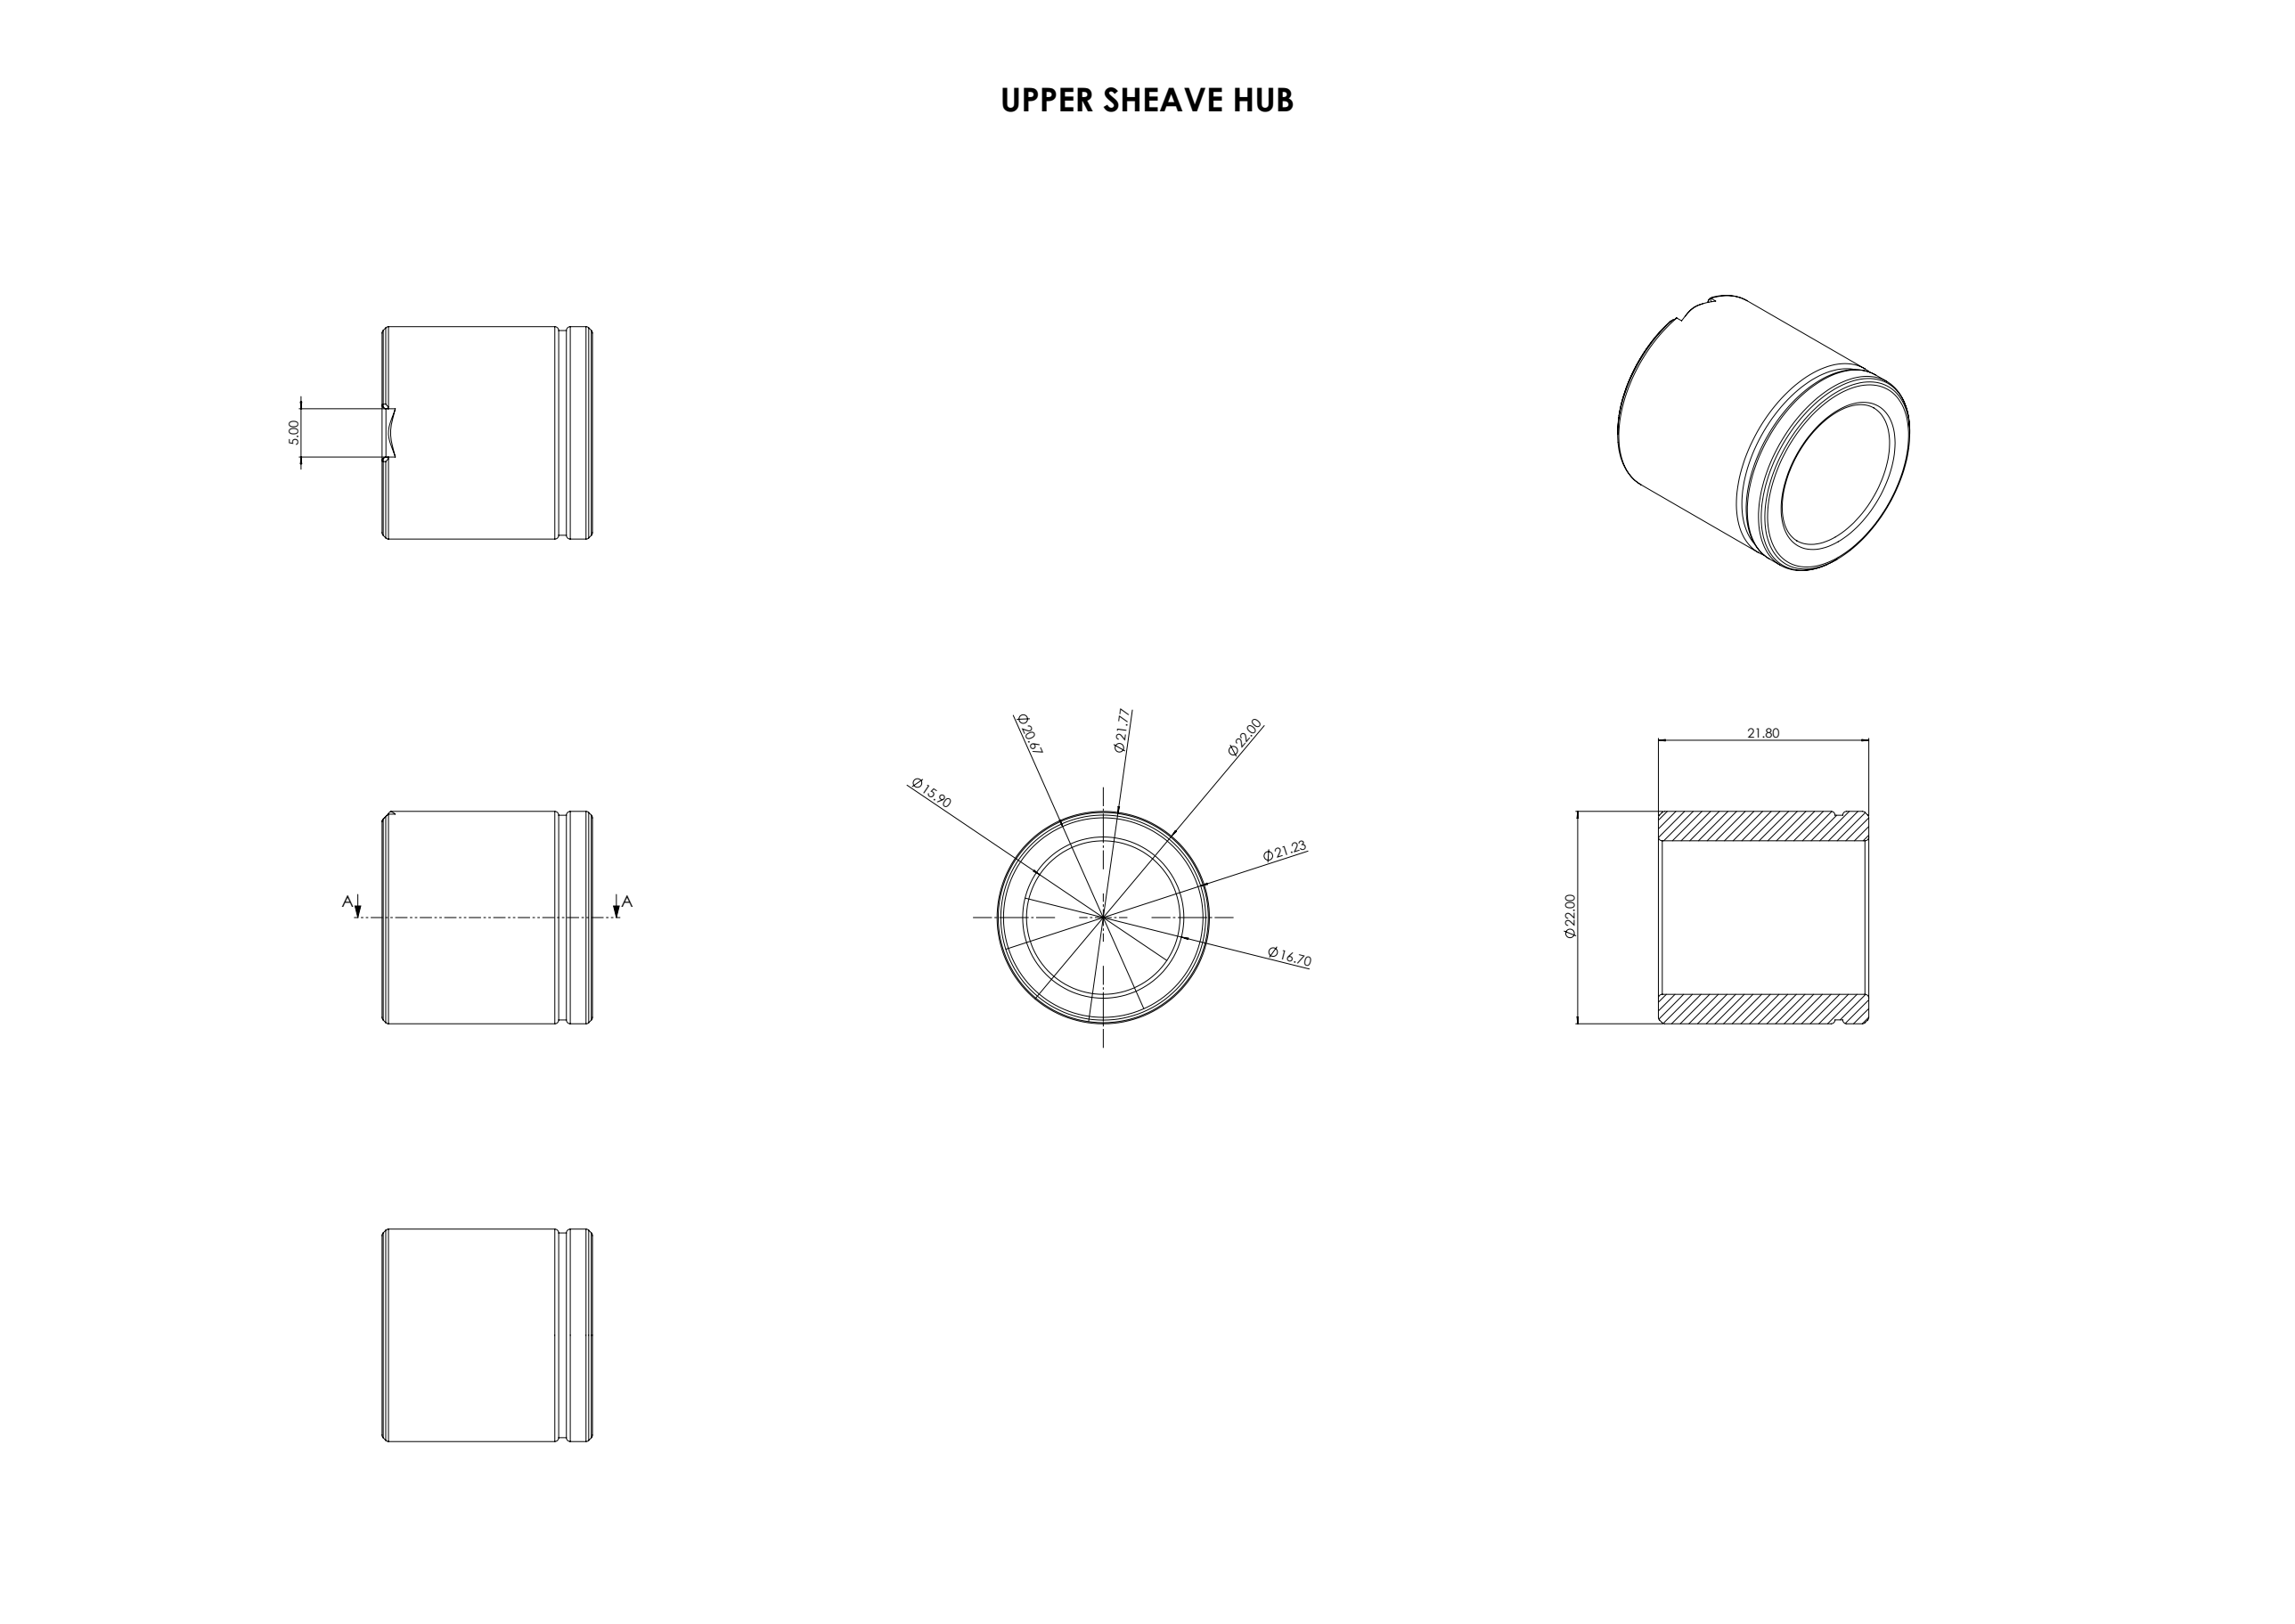
ISO-10303-21;
HEADER;
/* Generated by software containing ST-Developer
 * from STEP Tools, Inc. (www.steptools.com) 
 */

FILE_DESCRIPTION(
/* description */ (''),
/* implementation_level */ '2;1');

FILE_NAME(
/* name */ '05_Upper_Sheave_Hub.step',
/* time_stamp */ '2026-10-24T13:41:11-07:00',
/* author */ (''),
/* organization */ (''),
/* preprocessor_version */ 'ST-DEVELOPER v20.2',
/* originating_system */ 'Autodesk Translation Framework v15.15.0.0',
/* authorisation */ '');

FILE_SCHEMA (('AUTOMOTIVE_DESIGN { 1 0 10303 214 3 1 1 }'));
ENDSEC;

DATA;
#10=MECHANICAL_DESIGN_GEOMETRIC_PRESENTATION_REPRESENTATION('',(#125),#12813);
#77=SPHERICAL_SURFACE('',#4848,0.4);
#78=SPHERICAL_SURFACE('',#4850,0.4);
#79=SPHERICAL_SURFACE('',#4873,0.4);
#80=SPHERICAL_SURFACE('',#4876,0.4);
#92=CONICAL_SURFACE('',#4797,12.45,0.785398163397445);
#93=CONICAL_SURFACE('',#4806,12.45,0.785398163397445);
#94=CONICAL_SURFACE('',#4828,10.75,0.785398163397451);
#95=CONICAL_SURFACE('',#4840,10.75,0.785398163397451);
#105=SHAPE_REPRESENTATION_RELATIONSHIP('SRR','None',#12858,#115);
#115=ADVANCED_BREP_SHAPE_REPRESENTATION('',(#135),#12807);
#125=STYLED_ITEM('',(#12960),#135);
#135=MANIFOLD_SOLID_BREP('Body1',#4388);
#156=FACE_BOUND('',#779,.T.);
#157=FACE_BOUND('',#782,.T.);
#158=FACE_BOUND('',#811,.T.);
#206=PLANE('',#4804);
#207=PLANE('',#4808);
#208=PLANE('',#4816);
#209=PLANE('',#4817);
#210=PLANE('',#4818);
#211=PLANE('',#4819);
#212=PLANE('',#4820);
#213=PLANE('',#4852);
#214=PLANE('',#4855);
#215=PLANE('',#4862);
#216=PLANE('',#4872);
#217=PLANE('',#4884);
#277=TOROIDAL_SURFACE('',#4821,10.6,0.4);
#278=TOROIDAL_SURFACE('',#4831,10.6,0.4);
#279=TOROIDAL_SURFACE('',#4838,10.6,0.4);
#280=TOROIDAL_SURFACE('',#4844,10.3343145750508,0.4);
#281=TOROIDAL_SURFACE('',#4859,10.3343145750508,0.4);
#282=TOROIDAL_SURFACE('',#4864,8.35,0.4);
#283=TOROIDAL_SURFACE('',#4879,8.35,0.4);
#284=TOROIDAL_SURFACE('',#4881,8.35,0.4);
#319=B_SPLINE_SURFACE_WITH_KNOTS('',3,3,((#11947,#11948,#11949,#11950,#11951,
#11952,#11953,#11954,#11955,#11956,#11957,#11958,#11959),(#11960,#11961,
#11962,#11963,#11964,#11965,#11966,#11967,#11968,#11969,#11970,#11971,#11972),
(#11973,#11974,#11975,#11976,#11977,#11978,#11979,#11980,#11981,#11982,
#11983,#11984,#11985),(#11986,#11987,#11988,#11989,#11990,#11991,#11992,
#11993,#11994,#11995,#11996,#11997,#11998),(#11999,#12000,#12001,#12002,
#12003,#12004,#12005,#12006,#12007,#12008,#12009,#12010,#12011),(#12012,
#12013,#12014,#12015,#12016,#12017,#12018,#12019,#12020,#12021,#12022,#12023,
#12024),(#12025,#12026,#12027,#12028,#12029,#12030,#12031,#12032,#12033,
#12034,#12035,#12036,#12037)),.UNSPECIFIED.,.F.,.F.,.F.,(4,1,1,1,4),(4,
1,1,1,1,1,1,1,1,1,4),(0.,0.285714285714286,0.571428571428571,0.785714285714286,
1.),(-0.510305664677257,-0.435654171543958,-0.361002678410658,-0.323676931844009,
-0.305014058560684,-0.286351185277359,-0.267688311994034,-0.211699692144059,
-0.13704819901076,-0.0623967058774603,0.0122547872558393),.UNSPECIFIED.);
#320=B_SPLINE_SURFACE_WITH_KNOTS('',3,3,((#12242,#12243,#12244,#12245),
(#12246,#12247,#12248,#12249),(#12250,#12251,#12252,#12253),(#12254,#12255,
#12256,#12257),(#12258,#12259,#12260,#12261),(#12262,#12263,#12264,#12265)),
 .UNSPECIFIED.,.F.,.F.,.F.,(4,1,1,4),(4,4),(0.,0.285714285714286,0.571428571428571,
1.),(0.,0.0695988259914621),.UNSPECIFIED.);
#321=B_SPLINE_SURFACE_WITH_KNOTS('',3,3,((#12295,#12296,#12297,#12298),
(#12299,#12300,#12301,#12302),(#12303,#12304,#12305,#12306),(#12307,#12308,
#12309,#12310),(#12311,#12312,#12313,#12314)),.UNSPECIFIED.,.F.,.F.,.F.,
(4,1,4),(4,4),(0.248288368736695,0.460547516100694,0.743559712586026),(1.50567154478811,
1.5257178645514),.UNSPECIFIED.);
#322=B_SPLINE_SURFACE_WITH_KNOTS('',3,3,((#12315,#12316,#12317,#12318),
(#12319,#12320,#12321,#12322),(#12323,#12324,#12325,#12326),(#12327,#12328,
#12329,#12330),(#12331,#12332,#12333,#12334)),.UNSPECIFIED.,.F.,.F.,.F.,
(4,1,4),(4,4),(0.248288368736683,0.460547516100081,0.743559712584612),(0.999225034210935,
1.01926765266779),.UNSPECIFIED.);
#323=B_SPLINE_SURFACE_WITH_KNOTS('',3,3,((#12395,#12396,#12397,#12398),
(#12399,#12400,#12401,#12402),(#12403,#12404,#12405,#12406),(#12407,#12408,
#12409,#12410),(#12411,#12412,#12413,#12414),(#12415,#12416,#12417,#12418)),
 .UNSPECIFIED.,.F.,.F.,.F.,(4,1,1,4),(4,4),(0.,0.285714285714286,0.571428571428571,
1.),(0.096109917502246,0.165708743493706),.UNSPECIFIED.);
#491=FACE_OUTER_BOUND('',#776,.T.);
#492=FACE_OUTER_BOUND('',#777,.T.);
#493=FACE_OUTER_BOUND('',#778,.T.);
#494=FACE_OUTER_BOUND('',#780,.T.);
#495=FACE_OUTER_BOUND('',#781,.T.);
#496=FACE_OUTER_BOUND('',#783,.T.);
#497=FACE_OUTER_BOUND('',#784,.T.);
#498=FACE_OUTER_BOUND('',#785,.T.);
#499=FACE_OUTER_BOUND('',#786,.T.);
#500=FACE_OUTER_BOUND('',#787,.T.);
#501=FACE_OUTER_BOUND('',#788,.T.);
#502=FACE_OUTER_BOUND('',#789,.T.);
#503=FACE_OUTER_BOUND('',#790,.T.);
#504=FACE_OUTER_BOUND('',#791,.T.);
#505=FACE_OUTER_BOUND('',#792,.T.);
#506=FACE_OUTER_BOUND('',#793,.T.);
#507=FACE_OUTER_BOUND('',#794,.T.);
#508=FACE_OUTER_BOUND('',#795,.T.);
#509=FACE_OUTER_BOUND('',#796,.T.);
#510=FACE_OUTER_BOUND('',#797,.T.);
#511=FACE_OUTER_BOUND('',#798,.T.);
#512=FACE_OUTER_BOUND('',#799,.T.);
#513=FACE_OUTER_BOUND('',#800,.T.);
#514=FACE_OUTER_BOUND('',#801,.T.);
#515=FACE_OUTER_BOUND('',#802,.T.);
#516=FACE_OUTER_BOUND('',#803,.T.);
#517=FACE_OUTER_BOUND('',#804,.T.);
#518=FACE_OUTER_BOUND('',#805,.T.);
#519=FACE_OUTER_BOUND('',#806,.T.);
#520=FACE_OUTER_BOUND('',#807,.T.);
#521=FACE_OUTER_BOUND('',#808,.T.);
#522=FACE_OUTER_BOUND('',#809,.T.);
#523=FACE_OUTER_BOUND('',#810,.T.);
#524=FACE_OUTER_BOUND('',#812,.T.);
#525=FACE_OUTER_BOUND('',#813,.T.);
#526=FACE_OUTER_BOUND('',#814,.T.);
#527=FACE_OUTER_BOUND('',#815,.T.);
#528=FACE_OUTER_BOUND('',#816,.T.);
#529=FACE_OUTER_BOUND('',#817,.T.);
#530=FACE_OUTER_BOUND('',#818,.T.);
#531=FACE_OUTER_BOUND('',#819,.T.);
#532=FACE_OUTER_BOUND('',#820,.T.);
#533=FACE_OUTER_BOUND('',#821,.T.);
#776=EDGE_LOOP('',(#3569,#3570,#3571,#3572,#3573));
#777=EDGE_LOOP('',(#3574,#3575,#3576,#3577,#3578,#3579));
#778=EDGE_LOOP('',(#3580));
#779=EDGE_LOOP('',(#3581));
#780=EDGE_LOOP('',(#3582,#3583,#3584,#3585,#3586));
#781=EDGE_LOOP('',(#3587));
#782=EDGE_LOOP('',(#3588));
#783=EDGE_LOOP('',(#3589,#3590,#3591,#3592));
#784=EDGE_LOOP('',(#3593,#3594,#3595,#3596));
#785=EDGE_LOOP('',(#3597,#3598,#3599));
#786=EDGE_LOOP('',(#3600,#3601,#3602));
#787=EDGE_LOOP('',(#3603,#3604,#3605));
#788=EDGE_LOOP('',(#3606,#3607,#3608));
#789=EDGE_LOOP('',(#3609,#3610,#3611,#3612,#3613,#3614,#3615,#3616,#3617,
#3618,#3619,#3620,#3621,#3622));
#790=EDGE_LOOP('',(#3623,#3624,#3625,#3626));
#791=EDGE_LOOP('',(#3627,#3628,#3629,#3630,#3631,#3632));
#792=EDGE_LOOP('',(#3633,#3634,#3635,#3636,#3637));
#793=EDGE_LOOP('',(#3638,#3639,#3640,#3641,#3642,#3643));
#794=EDGE_LOOP('',(#3644,#3645,#3646,#3647,#3648));
#795=EDGE_LOOP('',(#3649,#3650,#3651,#3652,#3653,#3654,#3655,#3656,#3657));
#796=EDGE_LOOP('',(#3658,#3659,#3660,#3661,#3662,#3663,#3664,#3665,#3666));
#797=EDGE_LOOP('',(#3667,#3668,#3669,#3670));
#798=EDGE_LOOP('',(#3671,#3672,#3673,#3674,#3675));
#799=EDGE_LOOP('',(#3676,#3677,#3678));
#800=EDGE_LOOP('',(#3679,#3680,#3681));
#801=EDGE_LOOP('',(#3682,#3683,#3684,#3685,#3686));
#802=EDGE_LOOP('',(#3687,#3688,#3689,#3690));
#803=EDGE_LOOP('',(#3691,#3692,#3693));
#804=EDGE_LOOP('',(#3694,#3695,#3696));
#805=EDGE_LOOP('',(#3697,#3698,#3699,#3700,#3701,#3702,#3703,#3704,#3705,
#3706,#3707,#3708,#3709,#3710));
#806=EDGE_LOOP('',(#3711,#3712,#3713,#3714));
#807=EDGE_LOOP('',(#3715,#3716,#3717,#3718));
#808=EDGE_LOOP('',(#3719,#3720,#3721,#3722));
#809=EDGE_LOOP('',(#3723,#3724,#3725,#3726,#3727));
#810=EDGE_LOOP('',(#3728));
#811=EDGE_LOOP('',(#3729));
#812=EDGE_LOOP('',(#3730,#3731,#3732,#3733,#3734));
#813=EDGE_LOOP('',(#3735,#3736,#3737,#3738,#3739,#3740,#3741,#3742,#3743));
#814=EDGE_LOOP('',(#3744,#3745,#3746,#3747,#3748,#3749,#3750,#3751,#3752,
#3753,#3754,#3755));
#815=EDGE_LOOP('',(#3756,#3757,#3758));
#816=EDGE_LOOP('',(#3759,#3760,#3761));
#817=EDGE_LOOP('',(#3762,#3763,#3764,#3765,#3766));
#818=EDGE_LOOP('',(#3767,#3768,#3769,#3770));
#819=EDGE_LOOP('',(#3771,#3772,#3773,#3774,#3775,#3776));
#820=EDGE_LOOP('',(#3777,#3778,#3779,#3780));
#821=EDGE_LOOP('',(#3781,#3782,#3783,#3784));
#1032=CIRCLE('',#4798,12.6);
#1033=CIRCLE('',#4799,12.6);
#1034=CIRCLE('',#4800,12.3);
#1035=CIRCLE('',#4802,12.6);
#1036=CIRCLE('',#4803,12.6);
#1037=CIRCLE('',#4805,10.6);
#1038=CIRCLE('',#4807,12.3);
#1039=CIRCLE('',#4809,11.);
#1040=CIRCLE('',#4811,10.5);
#1041=CIRCLE('',#4812,10.5);
#1042=CIRCLE('',#4814,10.5);
#1043=CIRCLE('',#4815,10.5);
#1044=CIRCLE('',#4822,10.8828427124746);
#1045=CIRCLE('',#4823,10.8828427124746);
#1046=CIRCLE('',#4824,0.4);
#1047=CIRCLE('',#4825,11.);
#1048=CIRCLE('',#4826,11.);
#1049=CIRCLE('',#4829,10.6171572875254);
#1050=CIRCLE('',#4830,10.6171572875254);
#1051=CIRCLE('',#4832,0.4);
#1052=CIRCLE('',#4833,11.);
#1053=CIRCLE('',#4834,11.);
#1054=CIRCLE('',#4836,11.);
#1055=CIRCLE('',#4837,11.);
#1056=CIRCLE('',#4839,10.8828427124746);
#1057=CIRCLE('',#4841,10.6171572875254);
#1058=CIRCLE('',#4842,0.4);
#1059=CIRCLE('',#4843,0.4);
#1060=CIRCLE('',#4845,0.400000000000002);
#1061=CIRCLE('',#4846,10.3343145750508);
#1062=CIRCLE('',#4847,0.4);
#1063=CIRCLE('',#4849,0.400000000000003);
#1064=CIRCLE('',#4851,0.400000000000003);
#1065=CIRCLE('',#4854,0.4);
#1066=CIRCLE('',#4856,8.35);
#1067=CIRCLE('',#4858,0.4);
#1068=CIRCLE('',#4860,10.3343145750508);
#1069=CIRCLE('',#4861,0.4);
#1070=CIRCLE('',#4863,8.35);
#1071=CIRCLE('',#4865,7.95);
#1072=CIRCLE('',#4866,7.95);
#1073=CIRCLE('',#4867,0.4);
#1074=CIRCLE('',#4869,7.95);
#1075=CIRCLE('',#4870,7.95);
#1076=CIRCLE('',#4871,7.95);
#1077=CIRCLE('',#4874,0.4);
#1078=CIRCLE('',#4875,0.4);
#1079=CIRCLE('',#4877,0.400000000000001);
#1080=CIRCLE('',#4878,0.4);
#1081=CIRCLE('',#4882,8.35);
#1236=LINE('',#11795,#1466);
#1237=LINE('',#11802,#1467);
#1238=LINE('',#11809,#1468);
#1239=LINE('',#11816,#1469);
#1240=LINE('',#11820,#1470);
#1241=LINE('',#11825,#1471);
#1242=LINE('',#11829,#1472);
#1243=LINE('',#11833,#1473);
#1244=LINE('',#11834,#1474);
#1245=LINE('',#11837,#1475);
#1246=LINE('',#11838,#1476);
#1247=LINE('',#11841,#1477);
#1248=LINE('',#11842,#1478);
#1249=LINE('',#11845,#1479);
#1250=LINE('',#11846,#1480);
#1251=LINE('',#11849,#1481);
#1252=LINE('',#11851,#1482);
#1253=LINE('',#11858,#1483);
#1254=LINE('',#11860,#1484);
#1255=LINE('',#11901,#1485);
#1256=LINE('',#11946,#1486);
#1257=LINE('',#12141,#1487);
#1258=LINE('',#12146,#1488);
#1259=LINE('',#12156,#1489);
#1260=LINE('',#12159,#1490);
#1261=LINE('',#12436,#1491);
#1262=LINE('',#12438,#1492);
#1263=LINE('',#12440,#1493);
#1264=LINE('',#12447,#1494);
#1265=LINE('',#12448,#1495);
#1266=LINE('',#12451,#1496);
#1267=LINE('',#12455,#1497);
#1268=LINE('',#12474,#1498);
#1269=LINE('',#12478,#1499);
#1270=LINE('',#12482,#1500);
#1271=LINE('',#12485,#1501);
#1466=VECTOR('',#5707,12.45);
#1467=VECTOR('',#5716,12.6);
#1468=VECTOR('',#5725,12.45);
#1469=VECTOR('',#5732,10.);
#1470=VECTOR('',#5735,10.);
#1471=VECTOR('',#5740,10.);
#1472=VECTOR('',#5743,10.);
#1473=VECTOR('',#5748,10.);
#1474=VECTOR('',#5749,10.);
#1475=VECTOR('',#5752,10.);
#1476=VECTOR('',#5753,10.);
#1477=VECTOR('',#5756,10.);
#1478=VECTOR('',#5757,10.);
#1479=VECTOR('',#5760,10.);
#1480=VECTOR('',#5761,10.);
#1481=VECTOR('',#5764,10.);
#1482=VECTOR('',#5765,10.);
#1483=VECTOR('',#5766,10.);
#1484=VECTOR('',#5767,10.);
#1485=VECTOR('',#5768,10.);
#1486=VECTOR('',#5769,10.);
#1487=VECTOR('',#5784,11.);
#1488=VECTOR('',#5789,10.75);
#1489=VECTOR('',#5802,11.);
#1490=VECTOR('',#5805,10.);
#1491=VECTOR('',#5838,10.);
#1492=VECTOR('',#5839,10.);
#1493=VECTOR('',#5840,10.);
#1494=VECTOR('',#5841,10.);
#1495=VECTOR('',#5842,10.);
#1496=VECTOR('',#5845,10.);
#1497=VECTOR('',#5850,10.);
#1498=VECTOR('',#5877,7.95);
#1499=VECTOR('',#5880,10.);
#1500=VECTOR('',#5883,10.);
#1501=VECTOR('',#5888,10.);
#1723=B_SPLINE_CURVE_WITH_KNOTS('',3,(#11853,#11854,#11855,#11856),
 .UNSPECIFIED.,.F.,.F.,(4,4),(-0.0736302548927899,-0.0606102871491874),
 .UNSPECIFIED.);
#1724=B_SPLINE_CURVE_WITH_KNOTS('',3,(#11862,#11863,#11864,#11865),
 .UNSPECIFIED.,.F.,.F.,(4,4),(-0.0535503409172659,0.),.UNSPECIFIED.);
#1725=B_SPLINE_CURVE_WITH_KNOTS('',3,(#11867,#11868,#11869,#11870,#11871,
#11872,#11873,#11874,#11875,#11876,#11877,#11878,#11879,#11880,#11881,#11882,
#11883,#11884,#11885,#11886,#11887,#11888,#11889,#11890,#11891,#11892,#11893,
#11894),.UNSPECIFIED.,.F.,.F.,(4,3,3,3,3,3,3,3,3,4),(-0.0707543141709639,
-0.0639700558869814,-0.0618906129072222,-0.0551601393419019,-0.0506565173110961,
-0.0464091777054624,-0.039691133709109,-0.0329985150203425,-0.0311186796527011,
-0.0241191350787041),.UNSPECIFIED.);
#1726=B_SPLINE_CURVE_WITH_KNOTS('',3,(#11896,#11897,#11898,#11899),
 .UNSPECIFIED.,.F.,.F.,(4,4),(0.,0.00710537445304894),.UNSPECIFIED.);
#1727=B_SPLINE_CURVE_WITH_KNOTS('',3,(#11903,#11904,#11905,#11906,#11907,
#11908,#11909,#11910,#11911,#11912,#11913,#11914,#11915,#11916,#11917,#11918,
#11919,#11920,#11921,#11922,#11923,#11924,#11925,#11926,#11927,#11928,#11929,
#11930,#11931,#11932,#11933,#11934,#11935,#11936,#11937,#11938,#11939,#11940,
#11941,#11942,#11943,#11944,#11945),.UNSPECIFIED.,.F.,.F.,(4,3,3,3,3,3,
3,3,3,3,3,3,3,3,4),(0.,0.00580629857172819,0.011668120368983,0.0175829585474277,
0.0201349204647166,0.0268347020686461,0.0295682026475181,0.0365019513209761,
0.0408129765218727,0.0451592379215555,0.0520962433453293,0.0563360701356979,
0.0584849555420972,0.0655164894020243,0.0715864535936182),.UNSPECIFIED.);
#1728=B_SPLINE_CURVE_WITH_KNOTS('',3,(#12040,#12041,#12042,#12043,#12044,
#12045,#12046,#12047,#12048,#12049,#12050,#12051,#12052,#12053,#12054,#12055,
#12056,#12057,#12058,#12059,#12060,#12061,#12062,#12063,#12064,#12065,#12066,
#12067,#12068,#12069,#12070,#12071,#12072,#12073,#12074,#12075,#12076,#12077,
#12078,#12079,#12080,#12081,#12082,#12083,#12084,#12085),.UNSPECIFIED.,
 .F.,.F.,(4,3,3,3,3,3,3,3,3,3,3,3,3,3,3,4),(0.,0.00694526795998421,0.0139543072598735,
0.015291136260988,0.0172103975930811,0.0240884241491964,0.0308533616756733,
0.0340363892002112,0.0409613583285485,0.0476241304298719,0.0499527776364528,
0.0515655803640436,0.0584478624259065,0.0609496822139948,0.0675796538345217,
0.0717651027806449),.UNSPECIFIED.);
#1729=B_SPLINE_CURVE_WITH_KNOTS('',3,(#12086,#12087,#12088,#12089,#12090,
#12091,#12092,#12093,#12094,#12095,#12096,#12097,#12098),.UNSPECIFIED.,
 .F.,.F.,(4,1,1,1,1,1,1,1,1,1,4),(-0.0122547872558393,0.0623967058774603,
0.13704819901076,0.211699692144059,0.267688311994034,0.286351185277359,
0.305014058560684,0.323676931844009,0.361002678410658,0.435654171543958,
0.510305664677257),.UNSPECIFIED.);
#1730=B_SPLINE_CURVE_WITH_KNOTS('',3,(#12099,#12100,#12101,#12102,#12103,
#12104,#12105,#12106,#12107,#12108,#12109,#12110,#12111,#12112,#12113,#12114,
#12115,#12116,#12117,#12118,#12119,#12120,#12121,#12122,#12123,#12124,#12125,
#12126,#12127,#12128,#12129),.UNSPECIFIED.,.F.,.F.,(4,3,3,3,3,3,3,3,3,3,
4),(0.000383354128218201,0.0625597845796719,0.136949375128678,0.174144170403181,
0.192741568040432,0.211338965677684,0.229936363314935,0.28572855622669,
0.360118146775696,0.434507737324702,0.496685534539592),.UNSPECIFIED.);
#1731=B_SPLINE_CURVE_WITH_KNOTS('',3,(#12163,#12164,#12165,#12166),
 .UNSPECIFIED.,.F.,.F.,(4,4),(-0.00710537445449871,0.),.UNSPECIFIED.);
#1732=B_SPLINE_CURVE_WITH_KNOTS('',3,(#12168,#12169,#12170,#12171),
 .UNSPECIFIED.,.F.,.F.,(4,4),(-0.0196379557516152,-0.000110621155015422),
 .UNSPECIFIED.);
#1733=B_SPLINE_CURVE_WITH_KNOTS('',3,(#12173,#12174,#12175,#12176,#12177,
#12178,#12179,#12180,#12181,#12182,#12183,#12184,#12185,#12186,#12187,#12188,
#12189,#12190,#12191,#12192,#12193,#12194,#12195,#12196,#12197),
 .UNSPECIFIED.,.F.,.F.,(4,3,3,3,3,3,3,3,4),(-0.0420242349144714,-0.034244024011145,
-0.0304445564291344,-0.0224018409775603,-0.0210691966450077,-0.0115168785817897,
-0.00144892293139089,0.,0.000288034171025875),.UNSPECIFIED.);
#1734=B_SPLINE_CURVE_WITH_KNOTS('',3,(#12201,#12202,#12203,#12204,#12205,
#12206,#12207,#12208,#12209,#12210,#12211,#12212,#12213,#12214,#12215,#12216,
#12217,#12218,#12219,#12220,#12221,#12222,#12223,#12224,#12225),
 .UNSPECIFIED.,.F.,.F.,(4,3,3,3,3,3,3,3,4),(-0.0422600918508368,-0.0419734950304658,
-0.0314914666110231,-0.021986817507206,-0.0210094381915805,-0.01300685760943,
-0.0116808634569233,-0.00393947746920935,-0.000158970042657082),
 .UNSPECIFIED.);
#1735=B_SPLINE_CURVE_WITH_KNOTS('',3,(#12226,#12227,#12228,#12229),
 .UNSPECIFIED.,.F.,.F.,(4,4),(-0.328977585058273,-0.317010469451376),
 .UNSPECIFIED.);
#1736=B_SPLINE_CURVE_WITH_KNOTS('',3,(#12232,#12233,#12234,#12235),
 .UNSPECIFIED.,.F.,.F.,(4,4),(0.,0.0383467777019652),.UNSPECIFIED.);
#1737=B_SPLINE_CURVE_WITH_KNOTS('',3,(#12238,#12239,#12240,#12241),
 .UNSPECIFIED.,.F.,.F.,(4,4),(0.127361965791744,0.165708743493706),
 .UNSPECIFIED.);
#1738=B_SPLINE_CURVE_WITH_KNOTS('',3,(#12266,#12267,#12268,#12269,#12270,
#12271,#12272,#12273,#12274,#12275,#12276,#12277,#12278,#12279,#12280,#12281,
#12282,#12283,#12284,#12285,#12286,#12287,#12288,#12289,#12290,#12291,#12292,
#12293),.UNSPECIFIED.,.F.,.F.,(4,3,3,3,3,3,3,3,3,4),(-0.103312994452742,
-0.0944972367595641,-0.0896726356037232,-0.081979706066035,-0.0758675452743191,
-0.0681010871890584,-0.0620124392214268,-0.0585654250906251,-0.0490657070288485,
-0.0435218377980582),.UNSPECIFIED.);
#1739=B_SPLINE_CURVE_WITH_KNOTS('',3,(#12336,#12337,#12338,#12339,#12340,
#12341,#12342,#12343,#12344,#12345,#12346,#12347,#12348,#12349,#12350,#12351,
#12352,#12353,#12354,#12355,#12356,#12357,#12358,#12359,#12360,#12361,#12362,
#12363,#12364,#12365,#12366),.UNSPECIFIED.,.F.,.F.,(4,3,3,3,3,3,3,3,3,3,
4),(-0.0462738036441523,-0.0389589150096727,-0.0346312122739206,-0.0286583377057116,
-0.0230059035179827,-0.0212406883770576,-0.0202962772284038,-0.014379131563933,
-0.0105565993757205,-0.00393990817803328,0.),.UNSPECIFIED.);
#1740=B_SPLINE_CURVE_WITH_KNOTS('',3,(#12367,#12368,#12369,#12370,#12371,
#12372,#12373,#12374,#12375,#12376,#12377,#12378,#12379,#12380,#12381,#12382,
#12383,#12384,#12385,#12386,#12387,#12388,#12389,#12390,#12391,#12392,#12393,
#12394),.UNSPECIFIED.,.F.,.F.,(4,3,3,3,3,3,3,3,3,4),(-0.070410764499354,
-0.0637409419809624,-0.0570604470106178,-0.0503274465588287,-0.0483425491955468,
-0.0438577936617308,-0.0371215088649918,-0.0325914562918353,-0.0258040649471257,
-0.023746438679814),.UNSPECIFIED.);
#1741=B_SPLINE_CURVE_WITH_KNOTS('',3,(#12421,#12422,#12423,#12424),
 .UNSPECIFIED.,.F.,.F.,(4,4),(-0.165708743493706,-0.112158402576443),
 .UNSPECIFIED.);
#1742=B_SPLINE_CURVE_WITH_KNOTS('',3,(#12442,#12443,#12444,#12445),
 .UNSPECIFIED.,.F.,.F.,(4,4),(-0.182084709739034,-0.169064741995431),
 .UNSPECIFIED.);
#1743=B_SPLINE_CURVE_WITH_KNOTS('',3,(#12494,#12495,#12496,#12497,#12498,
#12499,#12500,#12501,#12502,#12503),.UNSPECIFIED.,.F.,.F.,(4,2,2,2,4),(-0.000394703056647228,
0.,0.0306355392027269,0.0540522668896819,0.0684604040501524),
 .UNSPECIFIED.);
#1744=B_SPLINE_CURVE_WITH_KNOTS('',3,(#12505,#12506,#12507,#12508,#12509,
#12510,#12511,#12512,#12513,#12514),.UNSPECIFIED.,.F.,.F.,(4,2,2,2,4),(-0.147143178540475,
-0.1468201126579,-0.121744812771334,-0.102578136276002,-0.0907850237818083),
 .UNSPECIFIED.);
#1996=VERTEX_POINT('',#11790);
#1997=VERTEX_POINT('',#11791);
#1998=VERTEX_POINT('',#11794);
#1999=VERTEX_POINT('',#11798);
#2000=VERTEX_POINT('',#11799);
#2001=VERTEX_POINT('',#11804);
#2002=VERTEX_POINT('',#11807);
#2003=VERTEX_POINT('',#11811);
#2004=VERTEX_POINT('',#11814);
#2005=VERTEX_POINT('',#11815);
#2006=VERTEX_POINT('',#11817);
#2007=VERTEX_POINT('',#11819);
#2008=VERTEX_POINT('',#11823);
#2009=VERTEX_POINT('',#11824);
#2010=VERTEX_POINT('',#11826);
#2011=VERTEX_POINT('',#11828);
#2012=VERTEX_POINT('',#11832);
#2013=VERTEX_POINT('',#11836);
#2014=VERTEX_POINT('',#11840);
#2015=VERTEX_POINT('',#11844);
#2016=VERTEX_POINT('',#11848);
#2017=VERTEX_POINT('',#11850);
#2018=VERTEX_POINT('',#11852);
#2019=VERTEX_POINT('',#11857);
#2020=VERTEX_POINT('',#11859);
#2021=VERTEX_POINT('',#11861);
#2022=VERTEX_POINT('',#11866);
#2023=VERTEX_POINT('',#11895);
#2024=VERTEX_POINT('',#11900);
#2025=VERTEX_POINT('',#11902);
#2026=VERTEX_POINT('',#12038);
#2027=VERTEX_POINT('',#12039);
#2028=VERTEX_POINT('',#12131);
#2029=VERTEX_POINT('',#12132);
#2030=VERTEX_POINT('',#12135);
#2031=VERTEX_POINT('',#12137);
#2032=VERTEX_POINT('',#12143);
#2033=VERTEX_POINT('',#12144);
#2034=VERTEX_POINT('',#12149);
#2035=VERTEX_POINT('',#12151);
#2036=VERTEX_POINT('',#12155);
#2037=VERTEX_POINT('',#12157);
#2038=VERTEX_POINT('',#12162);
#2039=VERTEX_POINT('',#12167);
#2040=VERTEX_POINT('',#12172);
#2041=VERTEX_POINT('',#12198);
#2042=VERTEX_POINT('',#12200);
#2043=VERTEX_POINT('',#12231);
#2044=VERTEX_POINT('',#12236);
#2045=VERTEX_POINT('',#12335);
#2046=VERTEX_POINT('',#12419);
#2047=VERTEX_POINT('',#12426);
#2048=VERTEX_POINT('',#12428);
#2049=VERTEX_POINT('',#12437);
#2050=VERTEX_POINT('',#12439);
#2051=VERTEX_POINT('',#12441);
#2052=VERTEX_POINT('',#12446);
#2053=VERTEX_POINT('',#12450);
#2054=VERTEX_POINT('',#12454);
#2055=VERTEX_POINT('',#12460);
#2056=VERTEX_POINT('',#12464);
#2057=VERTEX_POINT('',#12467);
#2058=VERTEX_POINT('',#12468);
#2059=VERTEX_POINT('',#12473);
#2060=VERTEX_POINT('',#12475);
#2061=VERTEX_POINT('',#12477);
#2062=VERTEX_POINT('',#12479);
#2063=VERTEX_POINT('',#12481);
#2537=EDGE_CURVE('',#1996,#1997,#1032,.T.);
#2538=EDGE_CURVE('',#1997,#1996,#1033,.T.);
#2539=EDGE_CURVE('',#1996,#1998,#1236,.T.);
#2540=EDGE_CURVE('',#1998,#1998,#1034,.T.);
#2541=EDGE_CURVE('',#1999,#2000,#1035,.T.);
#2542=EDGE_CURVE('',#2000,#1999,#1036,.T.);
#2543=EDGE_CURVE('',#2000,#1997,#1237,.T.);
#2544=EDGE_CURVE('',#2001,#2001,#1037,.T.);
#2545=EDGE_CURVE('',#2002,#2002,#1038,.T.);
#2546=EDGE_CURVE('',#2002,#1999,#1238,.T.);
#2547=EDGE_CURVE('',#2003,#2003,#1039,.T.);
#2548=EDGE_CURVE('',#2004,#2005,#1239,.T.);
#2549=EDGE_CURVE('',#2006,#2004,#1040,.T.);
#2550=EDGE_CURVE('',#2007,#2006,#1240,.T.);
#2551=EDGE_CURVE('',#2007,#2005,#1041,.T.);
#2552=EDGE_CURVE('',#2008,#2009,#1241,.T.);
#2553=EDGE_CURVE('',#2008,#2010,#1042,.T.);
#2554=EDGE_CURVE('',#2011,#2010,#1242,.T.);
#2555=EDGE_CURVE('',#2009,#2011,#1043,.T.);
#2556=EDGE_CURVE('',#2005,#2012,#1243,.T.);
#2557=EDGE_CURVE('',#2012,#2007,#1244,.T.);
#2558=EDGE_CURVE('',#2013,#2008,#1245,.T.);
#2559=EDGE_CURVE('',#2010,#2013,#1246,.T.);
#2560=EDGE_CURVE('',#2014,#2004,#1247,.T.);
#2561=EDGE_CURVE('',#2006,#2014,#1248,.T.);
#2562=EDGE_CURVE('',#2009,#2015,#1249,.T.);
#2563=EDGE_CURVE('',#2015,#2011,#1250,.T.);
#2564=EDGE_CURVE('',#2016,#2013,#1251,.T.);
#2565=EDGE_CURVE('',#2017,#2016,#1252,.T.);
#2566=EDGE_CURVE('',#2018,#2017,#1723,.T.);
#2567=EDGE_CURVE('',#2019,#2018,#1253,.T.);
#2568=EDGE_CURVE('',#2020,#2019,#1254,.T.);
#2569=EDGE_CURVE('',#2021,#2020,#1724,.T.);
#2570=EDGE_CURVE('',#2021,#2022,#1725,.T.);
#2571=EDGE_CURVE('',#2023,#2022,#1726,.T.);
#2572=EDGE_CURVE('',#2023,#2024,#1255,.T.);
#2573=EDGE_CURVE('',#2025,#2024,#1727,.F.);
#2574=EDGE_CURVE('',#2015,#2025,#1256,.T.);
#2575=EDGE_CURVE('',#2026,#2027,#1728,.T.);
#2576=EDGE_CURVE('',#2026,#2025,#1729,.T.);
#2577=EDGE_CURVE('',#2024,#2027,#1730,.T.);
#2578=EDGE_CURVE('',#2028,#2029,#1044,.T.);
#2579=EDGE_CURVE('',#2029,#2028,#1045,.T.);
#2580=EDGE_CURVE('',#2028,#2030,#1046,.T.);
#2581=EDGE_CURVE('',#2030,#2031,#1047,.T.);
#2582=EDGE_CURVE('',#2031,#2030,#1048,.T.);
#2583=EDGE_CURVE('',#2031,#2003,#1257,.T.);
#2584=EDGE_CURVE('',#2032,#2033,#1049,.T.);
#2585=EDGE_CURVE('',#2032,#2029,#1258,.T.);
#2586=EDGE_CURVE('',#2033,#2032,#1050,.T.);
#2587=EDGE_CURVE('',#2001,#2034,#1051,.T.);
#2588=EDGE_CURVE('',#2034,#2035,#1052,.T.);
#2589=EDGE_CURVE('',#2035,#2034,#1053,.T.);
#2590=EDGE_CURVE('',#2035,#2036,#1259,.T.);
#2591=EDGE_CURVE('',#2037,#2036,#1054,.T.);
#2592=EDGE_CURVE('',#2027,#2037,#1260,.T.);
#2593=EDGE_CURVE('',#2036,#2023,#1055,.T.);
#2594=EDGE_CURVE('',#2038,#2037,#1731,.T.);
#2595=EDGE_CURVE('',#2022,#2039,#1732,.T.);
#2596=EDGE_CURVE('',#2039,#2040,#1733,.T.);
#2597=EDGE_CURVE('',#2040,#2041,#1056,.T.);
#2598=EDGE_CURVE('',#2041,#2042,#1734,.T.);
#2599=EDGE_CURVE('',#2042,#2038,#1735,.T.);
#2600=EDGE_CURVE('',#2043,#2040,#1736,.T.);
#2601=EDGE_CURVE('',#2044,#2043,#1057,.T.);
#2602=EDGE_CURVE('',#2041,#2044,#1737,.T.);
#2603=EDGE_CURVE('',#2021,#2039,#1738,.T.);
#2604=EDGE_CURVE('',#2020,#2043,#1058,.T.);
#2605=EDGE_CURVE('',#2045,#2042,#1739,.F.);
#2606=EDGE_CURVE('',#2038,#2045,#1740,.T.);
#2607=EDGE_CURVE('',#2044,#2046,#1059,.T.);
#2608=EDGE_CURVE('',#2046,#2045,#1741,.T.);
#2609=EDGE_CURVE('',#2043,#2047,#1060,.T.);
#2610=EDGE_CURVE('',#2047,#2048,#1061,.T.);
#2611=EDGE_CURVE('',#2048,#2044,#1062,.T.);
#2612=EDGE_CURVE('',#2048,#2046,#1063,.T.);
#2613=EDGE_CURVE('',#2020,#2047,#1064,.T.);
#2614=EDGE_CURVE('',#2026,#2014,#1261,.T.);
#2615=EDGE_CURVE('',#2049,#2046,#1262,.T.);
#2616=EDGE_CURVE('',#2050,#2049,#1263,.T.);
#2617=EDGE_CURVE('',#2051,#2050,#1742,.T.);
#2618=EDGE_CURVE('',#2052,#2051,#1264,.T.);
#2619=EDGE_CURVE('',#2012,#2052,#1265,.T.);
#2620=EDGE_CURVE('',#2048,#2053,#1266,.T.);
#2621=EDGE_CURVE('',#2053,#2049,#1065,.F.);
#2622=EDGE_CURVE('',#2054,#2047,#1267,.T.);
#2623=EDGE_CURVE('',#2053,#2054,#1066,.T.);
#2624=EDGE_CURVE('',#2019,#2054,#1067,.F.);
#2625=EDGE_CURVE('',#2055,#2055,#1068,.T.);
#2626=EDGE_CURVE('',#2055,#2033,#1069,.T.);
#2627=EDGE_CURVE('',#2056,#2056,#1070,.T.);
#2628=EDGE_CURVE('',#2057,#2058,#1071,.T.);
#2629=EDGE_CURVE('',#2058,#2057,#1072,.T.);
#2630=EDGE_CURVE('',#2057,#2056,#1073,.T.);
#2631=EDGE_CURVE('',#2058,#2059,#1268,.T.);
#2632=EDGE_CURVE('',#2060,#2059,#1074,.T.);
#2633=EDGE_CURVE('',#2061,#2060,#1269,.T.);
#2634=EDGE_CURVE('',#2062,#2061,#1075,.T.);
#2635=EDGE_CURVE('',#2063,#2062,#1270,.T.);
#2636=EDGE_CURVE('',#2059,#2063,#1076,.T.);
#2637=EDGE_CURVE('',#2052,#2016,#1271,.T.);
#2638=EDGE_CURVE('',#2049,#2063,#1077,.F.);
#2639=EDGE_CURVE('',#2063,#2053,#1078,.F.);
#2640=EDGE_CURVE('',#2060,#2019,#1079,.F.);
#2641=EDGE_CURVE('',#2054,#2060,#1080,.F.);
#2642=EDGE_CURVE('',#2062,#2050,#1743,.T.);
#2643=EDGE_CURVE('',#2061,#2018,#1744,.T.);
#2644=EDGE_CURVE('',#2017,#2051,#1081,.T.);
#3569=ORIENTED_EDGE('',*,*,#2537,.T.);
#3570=ORIENTED_EDGE('',*,*,#2538,.T.);
#3571=ORIENTED_EDGE('',*,*,#2539,.T.);
#3572=ORIENTED_EDGE('',*,*,#2540,.T.);
#3573=ORIENTED_EDGE('',*,*,#2539,.F.);
#3574=ORIENTED_EDGE('',*,*,#2541,.F.);
#3575=ORIENTED_EDGE('',*,*,#2542,.F.);
#3576=ORIENTED_EDGE('',*,*,#2543,.T.);
#3577=ORIENTED_EDGE('',*,*,#2537,.F.);
#3578=ORIENTED_EDGE('',*,*,#2538,.F.);
#3579=ORIENTED_EDGE('',*,*,#2543,.F.);
#3580=ORIENTED_EDGE('',*,*,#2540,.F.);
#3581=ORIENTED_EDGE('',*,*,#2544,.T.);
#3582=ORIENTED_EDGE('',*,*,#2545,.T.);
#3583=ORIENTED_EDGE('',*,*,#2546,.T.);
#3584=ORIENTED_EDGE('',*,*,#2541,.T.);
#3585=ORIENTED_EDGE('',*,*,#2542,.T.);
#3586=ORIENTED_EDGE('',*,*,#2546,.F.);
#3587=ORIENTED_EDGE('',*,*,#2545,.F.);
#3588=ORIENTED_EDGE('',*,*,#2547,.T.);
#3589=ORIENTED_EDGE('',*,*,#2548,.F.);
#3590=ORIENTED_EDGE('',*,*,#2549,.F.);
#3591=ORIENTED_EDGE('',*,*,#2550,.F.);
#3592=ORIENTED_EDGE('',*,*,#2551,.T.);
#3593=ORIENTED_EDGE('',*,*,#2552,.F.);
#3594=ORIENTED_EDGE('',*,*,#2553,.T.);
#3595=ORIENTED_EDGE('',*,*,#2554,.F.);
#3596=ORIENTED_EDGE('',*,*,#2555,.F.);
#3597=ORIENTED_EDGE('',*,*,#2556,.F.);
#3598=ORIENTED_EDGE('',*,*,#2551,.F.);
#3599=ORIENTED_EDGE('',*,*,#2557,.F.);
#3600=ORIENTED_EDGE('',*,*,#2558,.F.);
#3601=ORIENTED_EDGE('',*,*,#2559,.F.);
#3602=ORIENTED_EDGE('',*,*,#2553,.F.);
#3603=ORIENTED_EDGE('',*,*,#2560,.F.);
#3604=ORIENTED_EDGE('',*,*,#2561,.F.);
#3605=ORIENTED_EDGE('',*,*,#2549,.T.);
#3606=ORIENTED_EDGE('',*,*,#2562,.F.);
#3607=ORIENTED_EDGE('',*,*,#2555,.T.);
#3608=ORIENTED_EDGE('',*,*,#2563,.F.);
#3609=ORIENTED_EDGE('',*,*,#2563,.T.);
#3610=ORIENTED_EDGE('',*,*,#2554,.T.);
#3611=ORIENTED_EDGE('',*,*,#2559,.T.);
#3612=ORIENTED_EDGE('',*,*,#2564,.F.);
#3613=ORIENTED_EDGE('',*,*,#2565,.F.);
#3614=ORIENTED_EDGE('',*,*,#2566,.F.);
#3615=ORIENTED_EDGE('',*,*,#2567,.F.);
#3616=ORIENTED_EDGE('',*,*,#2568,.F.);
#3617=ORIENTED_EDGE('',*,*,#2569,.F.);
#3618=ORIENTED_EDGE('',*,*,#2570,.T.);
#3619=ORIENTED_EDGE('',*,*,#2571,.F.);
#3620=ORIENTED_EDGE('',*,*,#2572,.T.);
#3621=ORIENTED_EDGE('',*,*,#2573,.F.);
#3622=ORIENTED_EDGE('',*,*,#2574,.F.);
#3623=ORIENTED_EDGE('',*,*,#2575,.F.);
#3624=ORIENTED_EDGE('',*,*,#2576,.T.);
#3625=ORIENTED_EDGE('',*,*,#2573,.T.);
#3626=ORIENTED_EDGE('',*,*,#2577,.T.);
#3627=ORIENTED_EDGE('',*,*,#2578,.T.);
#3628=ORIENTED_EDGE('',*,*,#2579,.T.);
#3629=ORIENTED_EDGE('',*,*,#2580,.T.);
#3630=ORIENTED_EDGE('',*,*,#2581,.T.);
#3631=ORIENTED_EDGE('',*,*,#2582,.T.);
#3632=ORIENTED_EDGE('',*,*,#2580,.F.);
#3633=ORIENTED_EDGE('',*,*,#2582,.F.);
#3634=ORIENTED_EDGE('',*,*,#2583,.T.);
#3635=ORIENTED_EDGE('',*,*,#2547,.F.);
#3636=ORIENTED_EDGE('',*,*,#2583,.F.);
#3637=ORIENTED_EDGE('',*,*,#2581,.F.);
#3638=ORIENTED_EDGE('',*,*,#2584,.F.);
#3639=ORIENTED_EDGE('',*,*,#2585,.T.);
#3640=ORIENTED_EDGE('',*,*,#2578,.F.);
#3641=ORIENTED_EDGE('',*,*,#2579,.F.);
#3642=ORIENTED_EDGE('',*,*,#2585,.F.);
#3643=ORIENTED_EDGE('',*,*,#2586,.F.);
#3644=ORIENTED_EDGE('',*,*,#2544,.F.);
#3645=ORIENTED_EDGE('',*,*,#2587,.T.);
#3646=ORIENTED_EDGE('',*,*,#2588,.T.);
#3647=ORIENTED_EDGE('',*,*,#2589,.T.);
#3648=ORIENTED_EDGE('',*,*,#2587,.F.);
#3649=ORIENTED_EDGE('',*,*,#2589,.F.);
#3650=ORIENTED_EDGE('',*,*,#2590,.T.);
#3651=ORIENTED_EDGE('',*,*,#2591,.F.);
#3652=ORIENTED_EDGE('',*,*,#2592,.F.);
#3653=ORIENTED_EDGE('',*,*,#2577,.F.);
#3654=ORIENTED_EDGE('',*,*,#2572,.F.);
#3655=ORIENTED_EDGE('',*,*,#2593,.F.);
#3656=ORIENTED_EDGE('',*,*,#2590,.F.);
#3657=ORIENTED_EDGE('',*,*,#2588,.F.);
#3658=ORIENTED_EDGE('',*,*,#2594,.T.);
#3659=ORIENTED_EDGE('',*,*,#2591,.T.);
#3660=ORIENTED_EDGE('',*,*,#2593,.T.);
#3661=ORIENTED_EDGE('',*,*,#2571,.T.);
#3662=ORIENTED_EDGE('',*,*,#2595,.T.);
#3663=ORIENTED_EDGE('',*,*,#2596,.T.);
#3664=ORIENTED_EDGE('',*,*,#2597,.T.);
#3665=ORIENTED_EDGE('',*,*,#2598,.T.);
#3666=ORIENTED_EDGE('',*,*,#2599,.T.);
#3667=ORIENTED_EDGE('',*,*,#2597,.F.);
#3668=ORIENTED_EDGE('',*,*,#2600,.F.);
#3669=ORIENTED_EDGE('',*,*,#2601,.F.);
#3670=ORIENTED_EDGE('',*,*,#2602,.F.);
#3671=ORIENTED_EDGE('',*,*,#2596,.F.);
#3672=ORIENTED_EDGE('',*,*,#2603,.F.);
#3673=ORIENTED_EDGE('',*,*,#2569,.T.);
#3674=ORIENTED_EDGE('',*,*,#2604,.T.);
#3675=ORIENTED_EDGE('',*,*,#2600,.T.);
#3676=ORIENTED_EDGE('',*,*,#2595,.F.);
#3677=ORIENTED_EDGE('',*,*,#2570,.F.);
#3678=ORIENTED_EDGE('',*,*,#2603,.T.);
#3679=ORIENTED_EDGE('',*,*,#2599,.F.);
#3680=ORIENTED_EDGE('',*,*,#2605,.F.);
#3681=ORIENTED_EDGE('',*,*,#2606,.F.);
#3682=ORIENTED_EDGE('',*,*,#2598,.F.);
#3683=ORIENTED_EDGE('',*,*,#2602,.T.);
#3684=ORIENTED_EDGE('',*,*,#2607,.T.);
#3685=ORIENTED_EDGE('',*,*,#2608,.T.);
#3686=ORIENTED_EDGE('',*,*,#2605,.T.);
#3687=ORIENTED_EDGE('',*,*,#2609,.T.);
#3688=ORIENTED_EDGE('',*,*,#2610,.T.);
#3689=ORIENTED_EDGE('',*,*,#2611,.T.);
#3690=ORIENTED_EDGE('',*,*,#2601,.T.);
#3691=ORIENTED_EDGE('',*,*,#2611,.F.);
#3692=ORIENTED_EDGE('',*,*,#2612,.T.);
#3693=ORIENTED_EDGE('',*,*,#2607,.F.);
#3694=ORIENTED_EDGE('',*,*,#2604,.F.);
#3695=ORIENTED_EDGE('',*,*,#2613,.T.);
#3696=ORIENTED_EDGE('',*,*,#2609,.F.);
#3697=ORIENTED_EDGE('',*,*,#2561,.T.);
#3698=ORIENTED_EDGE('',*,*,#2614,.F.);
#3699=ORIENTED_EDGE('',*,*,#2575,.T.);
#3700=ORIENTED_EDGE('',*,*,#2592,.T.);
#3701=ORIENTED_EDGE('',*,*,#2594,.F.);
#3702=ORIENTED_EDGE('',*,*,#2606,.T.);
#3703=ORIENTED_EDGE('',*,*,#2608,.F.);
#3704=ORIENTED_EDGE('',*,*,#2615,.F.);
#3705=ORIENTED_EDGE('',*,*,#2616,.F.);
#3706=ORIENTED_EDGE('',*,*,#2617,.F.);
#3707=ORIENTED_EDGE('',*,*,#2618,.F.);
#3708=ORIENTED_EDGE('',*,*,#2619,.F.);
#3709=ORIENTED_EDGE('',*,*,#2557,.T.);
#3710=ORIENTED_EDGE('',*,*,#2550,.T.);
#3711=ORIENTED_EDGE('',*,*,#2612,.F.);
#3712=ORIENTED_EDGE('',*,*,#2620,.T.);
#3713=ORIENTED_EDGE('',*,*,#2621,.T.);
#3714=ORIENTED_EDGE('',*,*,#2615,.T.);
#3715=ORIENTED_EDGE('',*,*,#2610,.F.);
#3716=ORIENTED_EDGE('',*,*,#2622,.F.);
#3717=ORIENTED_EDGE('',*,*,#2623,.F.);
#3718=ORIENTED_EDGE('',*,*,#2620,.F.);
#3719=ORIENTED_EDGE('',*,*,#2613,.F.);
#3720=ORIENTED_EDGE('',*,*,#2568,.T.);
#3721=ORIENTED_EDGE('',*,*,#2624,.T.);
#3722=ORIENTED_EDGE('',*,*,#2622,.T.);
#3723=ORIENTED_EDGE('',*,*,#2625,.T.);
#3724=ORIENTED_EDGE('',*,*,#2626,.T.);
#3725=ORIENTED_EDGE('',*,*,#2586,.T.);
#3726=ORIENTED_EDGE('',*,*,#2584,.T.);
#3727=ORIENTED_EDGE('',*,*,#2626,.F.);
#3728=ORIENTED_EDGE('',*,*,#2625,.F.);
#3729=ORIENTED_EDGE('',*,*,#2627,.F.);
#3730=ORIENTED_EDGE('',*,*,#2628,.T.);
#3731=ORIENTED_EDGE('',*,*,#2629,.T.);
#3732=ORIENTED_EDGE('',*,*,#2630,.T.);
#3733=ORIENTED_EDGE('',*,*,#2627,.T.);
#3734=ORIENTED_EDGE('',*,*,#2630,.F.);
#3735=ORIENTED_EDGE('',*,*,#2628,.F.);
#3736=ORIENTED_EDGE('',*,*,#2629,.F.);
#3737=ORIENTED_EDGE('',*,*,#2631,.T.);
#3738=ORIENTED_EDGE('',*,*,#2632,.F.);
#3739=ORIENTED_EDGE('',*,*,#2633,.F.);
#3740=ORIENTED_EDGE('',*,*,#2634,.F.);
#3741=ORIENTED_EDGE('',*,*,#2635,.F.);
#3742=ORIENTED_EDGE('',*,*,#2636,.F.);
#3743=ORIENTED_EDGE('',*,*,#2631,.F.);
#3744=ORIENTED_EDGE('',*,*,#2562,.T.);
#3745=ORIENTED_EDGE('',*,*,#2574,.T.);
#3746=ORIENTED_EDGE('',*,*,#2576,.F.);
#3747=ORIENTED_EDGE('',*,*,#2614,.T.);
#3748=ORIENTED_EDGE('',*,*,#2560,.T.);
#3749=ORIENTED_EDGE('',*,*,#2548,.T.);
#3750=ORIENTED_EDGE('',*,*,#2556,.T.);
#3751=ORIENTED_EDGE('',*,*,#2619,.T.);
#3752=ORIENTED_EDGE('',*,*,#2637,.T.);
#3753=ORIENTED_EDGE('',*,*,#2564,.T.);
#3754=ORIENTED_EDGE('',*,*,#2558,.T.);
#3755=ORIENTED_EDGE('',*,*,#2552,.T.);
#3756=ORIENTED_EDGE('',*,*,#2638,.F.);
#3757=ORIENTED_EDGE('',*,*,#2621,.F.);
#3758=ORIENTED_EDGE('',*,*,#2639,.F.);
#3759=ORIENTED_EDGE('',*,*,#2640,.F.);
#3760=ORIENTED_EDGE('',*,*,#2641,.F.);
#3761=ORIENTED_EDGE('',*,*,#2624,.F.);
#3762=ORIENTED_EDGE('',*,*,#2639,.T.);
#3763=ORIENTED_EDGE('',*,*,#2623,.T.);
#3764=ORIENTED_EDGE('',*,*,#2641,.T.);
#3765=ORIENTED_EDGE('',*,*,#2632,.T.);
#3766=ORIENTED_EDGE('',*,*,#2636,.T.);
#3767=ORIENTED_EDGE('',*,*,#2616,.T.);
#3768=ORIENTED_EDGE('',*,*,#2638,.T.);
#3769=ORIENTED_EDGE('',*,*,#2635,.T.);
#3770=ORIENTED_EDGE('',*,*,#2642,.T.);
#3771=ORIENTED_EDGE('',*,*,#2634,.T.);
#3772=ORIENTED_EDGE('',*,*,#2643,.T.);
#3773=ORIENTED_EDGE('',*,*,#2566,.T.);
#3774=ORIENTED_EDGE('',*,*,#2644,.T.);
#3775=ORIENTED_EDGE('',*,*,#2617,.T.);
#3776=ORIENTED_EDGE('',*,*,#2642,.F.);
#3777=ORIENTED_EDGE('',*,*,#2633,.T.);
#3778=ORIENTED_EDGE('',*,*,#2640,.T.);
#3779=ORIENTED_EDGE('',*,*,#2567,.T.);
#3780=ORIENTED_EDGE('',*,*,#2643,.F.);
#3781=ORIENTED_EDGE('',*,*,#2644,.F.);
#3782=ORIENTED_EDGE('',*,*,#2565,.T.);
#3783=ORIENTED_EDGE('',*,*,#2637,.F.);
#3784=ORIENTED_EDGE('',*,*,#2618,.T.);
#4094=CYLINDRICAL_SURFACE('',#4801,12.6);
#4095=CYLINDRICAL_SURFACE('',#4810,10.5);
#4096=CYLINDRICAL_SURFACE('',#4813,10.5);
#4097=CYLINDRICAL_SURFACE('',#4827,11.);
#4098=CYLINDRICAL_SURFACE('',#4835,11.);
#4099=CYLINDRICAL_SURFACE('',#4853,0.4);
#4100=CYLINDRICAL_SURFACE('',#4857,0.4);
#4101=CYLINDRICAL_SURFACE('',#4868,7.95);
#4102=CYLINDRICAL_SURFACE('',#4880,0.4);
#4103=CYLINDRICAL_SURFACE('',#4883,0.4);
#4281=ADVANCED_FACE('',(#491),#92,.T.);
#4282=ADVANCED_FACE('',(#492),#4094,.T.);
#4283=ADVANCED_FACE('',(#493,#156),#206,.T.);
#4284=ADVANCED_FACE('',(#494),#93,.T.);
#4285=ADVANCED_FACE('',(#495,#157),#207,.T.);
#4286=ADVANCED_FACE('',(#496),#4095,.F.);
#4287=ADVANCED_FACE('',(#497),#4096,.F.);
#4288=ADVANCED_FACE('',(#498),#208,.T.);
#4289=ADVANCED_FACE('',(#499),#209,.T.);
#4290=ADVANCED_FACE('',(#500),#210,.T.);
#4291=ADVANCED_FACE('',(#501),#211,.T.);
#4292=ADVANCED_FACE('',(#502),#212,.F.);
#4293=ADVANCED_FACE('',(#503),#319,.F.);
#4294=ADVANCED_FACE('',(#504),#277,.T.);
#4295=ADVANCED_FACE('',(#505),#4097,.T.);
#4296=ADVANCED_FACE('',(#506),#94,.T.);
#4297=ADVANCED_FACE('',(#507),#278,.T.);
#4298=ADVANCED_FACE('',(#508),#4098,.T.);
#4299=ADVANCED_FACE('',(#509),#279,.T.);
#4300=ADVANCED_FACE('',(#510),#95,.T.);
#4301=ADVANCED_FACE('',(#511),#320,.F.);
#4302=ADVANCED_FACE('',(#512),#321,.F.);
#4303=ADVANCED_FACE('',(#513),#322,.F.);
#4304=ADVANCED_FACE('',(#514),#323,.F.);
#4305=ADVANCED_FACE('',(#515),#280,.T.);
#4306=ADVANCED_FACE('',(#516),#77,.T.);
#4307=ADVANCED_FACE('',(#517),#78,.T.);
#4308=ADVANCED_FACE('',(#518),#213,.F.);
#4309=ADVANCED_FACE('',(#519),#4099,.T.);
#4310=ADVANCED_FACE('',(#520),#214,.T.);
#4311=ADVANCED_FACE('',(#521),#4100,.T.);
#4312=ADVANCED_FACE('',(#522),#281,.T.);
#4313=ADVANCED_FACE('',(#523,#158),#215,.T.);
#4314=ADVANCED_FACE('',(#524),#282,.T.);
#4315=ADVANCED_FACE('',(#525),#4101,.F.);
#4316=ADVANCED_FACE('',(#526),#216,.F.);
#4317=ADVANCED_FACE('',(#527),#79,.T.);
#4318=ADVANCED_FACE('',(#528),#80,.T.);
#4319=ADVANCED_FACE('',(#529),#283,.T.);
#4320=ADVANCED_FACE('',(#530),#4102,.T.);
#4321=ADVANCED_FACE('',(#531),#284,.T.);
#4322=ADVANCED_FACE('',(#532),#4103,.T.);
#4323=ADVANCED_FACE('',(#533),#217,.F.);
#4388=CLOSED_SHELL('',(#4281,#4282,#4283,#4284,#4285,#4286,#4287,#4288,
#4289,#4290,#4291,#4292,#4293,#4294,#4295,#4296,#4297,#4298,#4299,#4300,
#4301,#4302,#4303,#4304,#4305,#4306,#4307,#4308,#4309,#4310,#4311,#4312,
#4313,#4314,#4315,#4316,#4317,#4318,#4319,#4320,#4321,#4322,#4323));
#4796=AXIS2_PLACEMENT_3D('',#11788,#5699,#5700);
#4797=AXIS2_PLACEMENT_3D('',#11789,#5701,#5702);
#4798=AXIS2_PLACEMENT_3D('',#11792,#5703,#5704);
#4799=AXIS2_PLACEMENT_3D('',#11793,#5705,#5706);
#4800=AXIS2_PLACEMENT_3D('',#11796,#5708,#5709);
#4801=AXIS2_PLACEMENT_3D('',#11797,#5710,#5711);
#4802=AXIS2_PLACEMENT_3D('',#11800,#5712,#5713);
#4803=AXIS2_PLACEMENT_3D('',#11801,#5714,#5715);
#4804=AXIS2_PLACEMENT_3D('',#11803,#5717,#5718);
#4805=AXIS2_PLACEMENT_3D('',#11805,#5719,#5720);
#4806=AXIS2_PLACEMENT_3D('',#11806,#5721,#5722);
#4807=AXIS2_PLACEMENT_3D('',#11808,#5723,#5724);
#4808=AXIS2_PLACEMENT_3D('',#11810,#5726,#5727);
#4809=AXIS2_PLACEMENT_3D('',#11812,#5728,#5729);
#4810=AXIS2_PLACEMENT_3D('',#11813,#5730,#5731);
#4811=AXIS2_PLACEMENT_3D('',#11818,#5733,#5734);
#4812=AXIS2_PLACEMENT_3D('',#11821,#5736,#5737);
#4813=AXIS2_PLACEMENT_3D('',#11822,#5738,#5739);
#4814=AXIS2_PLACEMENT_3D('',#11827,#5741,#5742);
#4815=AXIS2_PLACEMENT_3D('',#11830,#5744,#5745);
#4816=AXIS2_PLACEMENT_3D('',#11831,#5746,#5747);
#4817=AXIS2_PLACEMENT_3D('',#11835,#5750,#5751);
#4818=AXIS2_PLACEMENT_3D('',#11839,#5754,#5755);
#4819=AXIS2_PLACEMENT_3D('',#11843,#5758,#5759);
#4820=AXIS2_PLACEMENT_3D('',#11847,#5762,#5763);
#4821=AXIS2_PLACEMENT_3D('',#12130,#5770,#5771);
#4822=AXIS2_PLACEMENT_3D('',#12133,#5772,#5773);
#4823=AXIS2_PLACEMENT_3D('',#12134,#5774,#5775);
#4824=AXIS2_PLACEMENT_3D('',#12136,#5776,#5777);
#4825=AXIS2_PLACEMENT_3D('',#12138,#5778,#5779);
#4826=AXIS2_PLACEMENT_3D('',#12139,#5780,#5781);
#4827=AXIS2_PLACEMENT_3D('',#12140,#5782,#5783);
#4828=AXIS2_PLACEMENT_3D('',#12142,#5785,#5786);
#4829=AXIS2_PLACEMENT_3D('',#12145,#5787,#5788);
#4830=AXIS2_PLACEMENT_3D('',#12147,#5790,#5791);
#4831=AXIS2_PLACEMENT_3D('',#12148,#5792,#5793);
#4832=AXIS2_PLACEMENT_3D('',#12150,#5794,#5795);
#4833=AXIS2_PLACEMENT_3D('',#12152,#5796,#5797);
#4834=AXIS2_PLACEMENT_3D('',#12153,#5798,#5799);
#4835=AXIS2_PLACEMENT_3D('',#12154,#5800,#5801);
#4836=AXIS2_PLACEMENT_3D('',#12158,#5803,#5804);
#4837=AXIS2_PLACEMENT_3D('',#12160,#5806,#5807);
#4838=AXIS2_PLACEMENT_3D('',#12161,#5808,#5809);
#4839=AXIS2_PLACEMENT_3D('',#12199,#5810,#5811);
#4840=AXIS2_PLACEMENT_3D('',#12230,#5812,#5813);
#4841=AXIS2_PLACEMENT_3D('',#12237,#5814,#5815);
#4842=AXIS2_PLACEMENT_3D('',#12294,#5816,#5817);
#4843=AXIS2_PLACEMENT_3D('',#12420,#5818,#5819);
#4844=AXIS2_PLACEMENT_3D('',#12425,#5820,#5821);
#4845=AXIS2_PLACEMENT_3D('',#12427,#5822,#5823);
#4846=AXIS2_PLACEMENT_3D('',#12429,#5824,#5825);
#4847=AXIS2_PLACEMENT_3D('',#12430,#5826,#5827);
#4848=AXIS2_PLACEMENT_3D('',#12431,#5828,#5829);
#4849=AXIS2_PLACEMENT_3D('',#12432,#5830,#5831);
#4850=AXIS2_PLACEMENT_3D('',#12433,#5832,#5833);
#4851=AXIS2_PLACEMENT_3D('',#12434,#5834,#5835);
#4852=AXIS2_PLACEMENT_3D('',#12435,#5836,#5837);
#4853=AXIS2_PLACEMENT_3D('',#12449,#5843,#5844);
#4854=AXIS2_PLACEMENT_3D('',#12452,#5846,#5847);
#4855=AXIS2_PLACEMENT_3D('',#12453,#5848,#5849);
#4856=AXIS2_PLACEMENT_3D('',#12456,#5851,#5852);
#4857=AXIS2_PLACEMENT_3D('',#12457,#5853,#5854);
#4858=AXIS2_PLACEMENT_3D('',#12458,#5855,#5856);
#4859=AXIS2_PLACEMENT_3D('',#12459,#5857,#5858);
#4860=AXIS2_PLACEMENT_3D('',#12461,#5859,#5860);
#4861=AXIS2_PLACEMENT_3D('',#12462,#5861,#5862);
#4862=AXIS2_PLACEMENT_3D('',#12463,#5863,#5864);
#4863=AXIS2_PLACEMENT_3D('',#12465,#5865,#5866);
#4864=AXIS2_PLACEMENT_3D('',#12466,#5867,#5868);
#4865=AXIS2_PLACEMENT_3D('',#12469,#5869,#5870);
#4866=AXIS2_PLACEMENT_3D('',#12470,#5871,#5872);
#4867=AXIS2_PLACEMENT_3D('',#12471,#5873,#5874);
#4868=AXIS2_PLACEMENT_3D('',#12472,#5875,#5876);
#4869=AXIS2_PLACEMENT_3D('',#12476,#5878,#5879);
#4870=AXIS2_PLACEMENT_3D('',#12480,#5881,#5882);
#4871=AXIS2_PLACEMENT_3D('',#12483,#5884,#5885);
#4872=AXIS2_PLACEMENT_3D('',#12484,#5886,#5887);
#4873=AXIS2_PLACEMENT_3D('',#12486,#5889,#5890);
#4874=AXIS2_PLACEMENT_3D('',#12487,#5891,#5892);
#4875=AXIS2_PLACEMENT_3D('',#12488,#5893,#5894);
#4876=AXIS2_PLACEMENT_3D('',#12489,#5895,#5896);
#4877=AXIS2_PLACEMENT_3D('',#12490,#5897,#5898);
#4878=AXIS2_PLACEMENT_3D('',#12491,#5899,#5900);
#4879=AXIS2_PLACEMENT_3D('',#12492,#5901,#5902);
#4880=AXIS2_PLACEMENT_3D('',#12493,#5903,#5904);
#4881=AXIS2_PLACEMENT_3D('',#12504,#5905,#5906);
#4882=AXIS2_PLACEMENT_3D('',#12515,#5907,#5908);
#4883=AXIS2_PLACEMENT_3D('',#12516,#5909,#5910);
#4884=AXIS2_PLACEMENT_3D('',#12517,#5911,#5912);
#5699=DIRECTION('axis',(0.,0.,1.));
#5700=DIRECTION('refdir',(1.,0.,0.));
#5701=DIRECTION('center_axis',(1.,0.,0.));
#5702=DIRECTION('ref_axis',(0.,-1.,0.));
#5703=DIRECTION('center_axis',(-1.,0.,0.));
#5704=DIRECTION('ref_axis',(0.,-1.,0.));
#5705=DIRECTION('center_axis',(-1.,0.,0.));
#5706=DIRECTION('ref_axis',(0.,-1.,0.));
#5707=DIRECTION('',(-0.70710678118655,-0.707106781186545,-8.6595605623549E-17));
#5708=DIRECTION('center_axis',(1.,0.,0.));
#5709=DIRECTION('ref_axis',(0.,-1.,0.));
#5710=DIRECTION('center_axis',(1.,0.,0.));
#5711=DIRECTION('ref_axis',(0.,1.,0.));
#5712=DIRECTION('center_axis',(1.,0.,0.));
#5713=DIRECTION('ref_axis',(0.,-1.,0.));
#5714=DIRECTION('center_axis',(1.,0.,0.));
#5715=DIRECTION('ref_axis',(0.,-1.,0.));
#5716=DIRECTION('',(-1.,0.,0.));
#5717=DIRECTION('center_axis',(-1.,0.,0.));
#5718=DIRECTION('ref_axis',(0.,0.,1.));
#5719=DIRECTION('center_axis',(1.,0.,0.));
#5720=DIRECTION('ref_axis',(0.,0.,-1.));
#5721=DIRECTION('center_axis',(-1.,0.,0.));
#5722=DIRECTION('ref_axis',(0.,-1.,0.));
#5723=DIRECTION('center_axis',(-1.,0.,0.));
#5724=DIRECTION('ref_axis',(0.,-1.,0.));
#5725=DIRECTION('',(-0.70710678118655,0.707106781186545,8.6595605623549E-17));
#5726=DIRECTION('center_axis',(1.,0.,0.));
#5727=DIRECTION('ref_axis',(0.,0.,-1.));
#5728=DIRECTION('center_axis',(-1.,0.,0.));
#5729=DIRECTION('ref_axis',(0.,-1.,1.83697019872103E-16));
#5730=DIRECTION('center_axis',(1.,0.,0.));
#5731=DIRECTION('ref_axis',(0.,1.,0.));
#5732=DIRECTION('',(1.,0.,0.));
#5733=DIRECTION('center_axis',(1.,0.,0.));
#5734=DIRECTION('ref_axis',(0.,0.,-1.));
#5735=DIRECTION('',(-1.,0.,0.));
#5736=DIRECTION('center_axis',(1.,0.,0.));
#5737=DIRECTION('ref_axis',(0.,0.,-1.));
#5738=DIRECTION('center_axis',(1.,0.,0.));
#5739=DIRECTION('ref_axis',(0.,1.,0.));
#5740=DIRECTION('',(-1.,0.,0.));
#5741=DIRECTION('center_axis',(1.,0.,0.));
#5742=DIRECTION('ref_axis',(0.,0.,-1.));
#5743=DIRECTION('',(1.,0.,0.));
#5744=DIRECTION('center_axis',(1.,0.,0.));
#5745=DIRECTION('ref_axis',(0.,0.,-1.));
#5746=DIRECTION('center_axis',(1.,0.,0.));
#5747=DIRECTION('ref_axis',(0.,0.,-1.));
#5748=DIRECTION('',(0.,0.,-1.));
#5749=DIRECTION('',(0.,-1.,0.));
#5750=DIRECTION('center_axis',(1.,0.,0.));
#5751=DIRECTION('ref_axis',(0.,0.,-1.));
#5752=DIRECTION('',(0.,0.,-1.));
#5753=DIRECTION('',(0.,1.,0.));
#5754=DIRECTION('center_axis',(-1.,0.,0.));
#5755=DIRECTION('ref_axis',(0.,0.,1.));
#5756=DIRECTION('',(0.,0.,1.));
#5757=DIRECTION('',(0.,1.,0.));
#5758=DIRECTION('center_axis',(-1.,0.,0.));
#5759=DIRECTION('ref_axis',(0.,0.,1.));
#5760=DIRECTION('',(0.,0.,1.));
#5761=DIRECTION('',(0.,-1.,0.));
#5762=DIRECTION('center_axis',(0.,0.,1.));
#5763=DIRECTION('ref_axis',(1.,0.,0.));
#5764=DIRECTION('',(-1.,0.,0.));
#5765=DIRECTION('',(0.,1.,0.));
#5766=DIRECTION('',(1.,0.,0.));
#5767=DIRECTION('',(0.,-1.,0.));
#5768=DIRECTION('',(1.,0.,0.));
#5769=DIRECTION('',(-1.,0.,0.));
#5770=DIRECTION('center_axis',(1.,0.,0.));
#5771=DIRECTION('ref_axis',(0.,0.,-1.));
#5772=DIRECTION('center_axis',(-1.,0.,0.));
#5773=DIRECTION('ref_axis',(0.,-1.,3.06161699786838E-17));
#5774=DIRECTION('center_axis',(-1.,0.,0.));
#5775=DIRECTION('ref_axis',(0.,-1.,3.06161699786838E-17));
#5776=DIRECTION('center_axis',(0.,-1.,-1.22464679914735E-16));
#5777=DIRECTION('ref_axis',(0.,-1.22464679914735E-16,1.));
#5778=DIRECTION('center_axis',(1.,0.,0.));
#5779=DIRECTION('ref_axis',(0.,-1.,1.83697019872103E-16));
#5780=DIRECTION('center_axis',(1.,0.,0.));
#5781=DIRECTION('ref_axis',(0.,-1.,1.83697019872103E-16));
#5782=DIRECTION('center_axis',(1.,0.,0.));
#5783=DIRECTION('ref_axis',(0.,1.,0.));
#5784=DIRECTION('',(-1.,0.,0.));
#5785=DIRECTION('center_axis',(-1.,0.,0.));
#5786=DIRECTION('ref_axis',(0.,1.,0.));
#5787=DIRECTION('center_axis',(1.,0.,0.));
#5788=DIRECTION('ref_axis',(0.,-1.,3.06161699786838E-17));
#5789=DIRECTION('',(-0.707106781186546,-0.707106781186549,-8.65956056235495E-17));
#5790=DIRECTION('center_axis',(1.,0.,0.));
#5791=DIRECTION('ref_axis',(0.,-1.,3.06161699786838E-17));
#5792=DIRECTION('center_axis',(1.,0.,0.));
#5793=DIRECTION('ref_axis',(0.,0.,-1.));
#5794=DIRECTION('center_axis',(0.,-1.,-1.22464679914735E-16));
#5795=DIRECTION('ref_axis',(0.,-1.22464679914735E-16,1.));
#5796=DIRECTION('center_axis',(1.,0.,0.));
#5797=DIRECTION('ref_axis',(0.,-1.,1.83697019872103E-16));
#5798=DIRECTION('center_axis',(1.,0.,0.));
#5799=DIRECTION('ref_axis',(0.,-1.,1.83697019872103E-16));
#5800=DIRECTION('center_axis',(1.,0.,0.));
#5801=DIRECTION('ref_axis',(0.,1.,0.));
#5802=DIRECTION('',(-1.,0.,0.));
#5803=DIRECTION('center_axis',(-1.,0.,0.));
#5804=DIRECTION('ref_axis',(0.,-1.,1.83697019872103E-16));
#5805=DIRECTION('',(-1.,0.,0.));
#5806=DIRECTION('center_axis',(-1.,0.,0.));
#5807=DIRECTION('ref_axis',(0.,-1.,1.83697019872103E-16));
#5808=DIRECTION('center_axis',(1.,0.,0.));
#5809=DIRECTION('ref_axis',(0.,-1.,-6.12323399573677E-17));
#5810=DIRECTION('center_axis',(1.,0.,0.));
#5811=DIRECTION('ref_axis',(0.,-1.,3.06161699786838E-17));
#5812=DIRECTION('center_axis',(1.,0.,0.));
#5813=DIRECTION('ref_axis',(0.,-1.,1.22464679914735E-16));
#5814=DIRECTION('center_axis',(-1.,0.,0.));
#5815=DIRECTION('ref_axis',(0.,-1.,3.06161699786838E-17));
#5816=DIRECTION('center_axis',(0.692464013941372,0.721452416584908,-7.14974227561921E-12));
#5817=DIRECTION('ref_axis',(-1.03250741290139E-11,0.,-1.));
#5818=DIRECTION('center_axis',(0.692464013941369,0.721452416584911,7.14974227561918E-12));
#5819=DIRECTION('ref_axis',(-0.70710678118655,0.678694795014786,-0.198427254226414));
#5820=DIRECTION('center_axis',(1.,0.,0.));
#5821=DIRECTION('ref_axis',(0.,-1.,-1.17055854380544E-13));
#5822=DIRECTION('center_axis',(3.44290678714761E-15,-0.280618514071671,
0.959819383821877));
#5823=DIRECTION('ref_axis',(-0.707106781186548,0.678694795014742,0.198427254226573));
#5824=DIRECTION('center_axis',(1.,0.,0.));
#5825=DIRECTION('ref_axis',(0.,-1.,1.83697019872103E-16));
#5826=DIRECTION('center_axis',(6.88581357429522E-15,-0.28061851407167,-0.959819383821877));
#5827=DIRECTION('ref_axis',(-1.,-5.55111512312578E-15,-5.55111512312578E-15));
#5828=DIRECTION('center_axis',(-0.371626520792815,0.147747632515864,-0.91655025292091));
#5829=DIRECTION('ref_axis',(-0.851707287237021,0.338613441842967,0.399919534244846));
#5830=DIRECTION('center_axis',(0.,1.,0.));
#5831=DIRECTION('ref_axis',(-0.707106781186545,0.,0.70710678118655));
#5832=DIRECTION('center_axis',(0.371626520793064,-0.147747632509487,-0.916550252921837));
#5833=DIRECTION('ref_axis',(-0.851707287242982,0.338613441830485,-0.39991953424272));
#5834=DIRECTION('center_axis',(0.,1.,0.));
#5835=DIRECTION('ref_axis',(-0.707106781186545,0.,-0.70710678118655));
#5836=DIRECTION('center_axis',(0.,0.,-1.));
#5837=DIRECTION('ref_axis',(-1.,0.,0.));
#5838=DIRECTION('',(1.,0.,0.));
#5839=DIRECTION('',(0.,1.,0.));
#5840=DIRECTION('',(-1.,0.,0.));
#5841=DIRECTION('',(0.,-1.,0.));
#5842=DIRECTION('',(1.,0.,0.));
#5843=DIRECTION('center_axis',(0.,1.,0.));
#5844=DIRECTION('ref_axis',(-0.70710678118654,0.,0.707106781186555));
#5845=DIRECTION('',(0.,-1.,0.));
#5846=DIRECTION('center_axis',(0.,-1.,0.));
#5847=DIRECTION('ref_axis',(-1.,0.,0.));
#5848=DIRECTION('center_axis',(-1.,0.,0.));
#5849=DIRECTION('ref_axis',(0.,0.,1.));
#5850=DIRECTION('',(0.,1.,0.));
#5851=DIRECTION('center_axis',(-1.,0.,0.));
#5852=DIRECTION('ref_axis',(0.,-1.,1.83697019872103E-16));
#5853=DIRECTION('center_axis',(0.,-1.,0.));
#5854=DIRECTION('ref_axis',(-0.70710678118654,0.,-0.707106781186555));
#5855=DIRECTION('center_axis',(0.,-1.,0.));
#5856=DIRECTION('ref_axis',(0.,0.,-1.));
#5857=DIRECTION('center_axis',(1.,0.,0.));
#5858=DIRECTION('ref_axis',(0.,0.,-1.));
#5859=DIRECTION('center_axis',(-1.,0.,0.));
#5860=DIRECTION('ref_axis',(0.,-1.,1.83697019872103E-16));
#5861=DIRECTION('center_axis',(0.,-1.,-1.22464679914735E-16));
#5862=DIRECTION('ref_axis',(0.,-1.22464679914735E-16,1.));
#5863=DIRECTION('center_axis',(1.,0.,0.));
#5864=DIRECTION('ref_axis',(0.,0.,-1.));
#5865=DIRECTION('center_axis',(1.,0.,0.));
#5866=DIRECTION('ref_axis',(0.,-1.,1.83697019872103E-16));
#5867=DIRECTION('center_axis',(1.,0.,0.));
#5868=DIRECTION('ref_axis',(0.,0.,-1.));
#5869=DIRECTION('center_axis',(-1.,0.,0.));
#5870=DIRECTION('ref_axis',(0.,-1.,1.83697019872103E-16));
#5871=DIRECTION('center_axis',(-1.,0.,0.));
#5872=DIRECTION('ref_axis',(0.,-1.,1.83697019872103E-16));
#5873=DIRECTION('center_axis',(0.,-1.,-1.22464679914735E-16));
#5874=DIRECTION('ref_axis',(0.,-1.22464679914735E-16,1.));
#5875=DIRECTION('center_axis',(1.,0.,0.));
#5876=DIRECTION('ref_axis',(0.,1.,0.));
#5877=DIRECTION('',(-1.,0.,0.));
#5878=DIRECTION('center_axis',(1.,0.,0.));
#5879=DIRECTION('ref_axis',(0.,-1.,1.83697019872103E-16));
#5880=DIRECTION('',(-1.,0.,0.));
#5881=DIRECTION('center_axis',(1.,0.,0.));
#5882=DIRECTION('ref_axis',(0.,1.,0.));
#5883=DIRECTION('',(1.,0.,0.));
#5884=DIRECTION('center_axis',(1.,0.,0.));
#5885=DIRECTION('ref_axis',(0.,-1.,1.83697019872103E-16));
#5886=DIRECTION('center_axis',(0.,1.,0.));
#5887=DIRECTION('ref_axis',(-1.,0.,0.));
#5888=DIRECTION('',(0.,0.,1.));
#5889=DIRECTION('center_axis',(0.290768000350851,-0.8729165634249,-0.391753293885871));
#5890=DIRECTION('ref_axis',(-0.520254270210838,-0.48786952487162,0.700941382020586));
#5891=DIRECTION('center_axis',(-1.,0.,0.));
#5892=DIRECTION('ref_axis',(0.,0.,1.));
#5893=DIRECTION('center_axis',(0.,0.347305389221559,0.937752081638672));
#5894=DIRECTION('ref_axis',(0.,-0.937752081638672,0.347305389221559));
#5895=DIRECTION('center_axis',(0.290768000350852,-0.872916563424899,0.391753293885873));
#5896=DIRECTION('ref_axis',(-0.520254270210838,-0.487869524871625,-0.700941382020582));
#5897=DIRECTION('center_axis',(-1.,0.,0.));
#5898=DIRECTION('ref_axis',(0.,-0.937752081638672,-0.347305389221556));
#5899=DIRECTION('center_axis',(0.,0.347305389221548,-0.937752081638676));
#5900=DIRECTION('ref_axis',(-1.,0.,0.));
#5901=DIRECTION('center_axis',(1.,0.,0.));
#5902=DIRECTION('ref_axis',(0.,-1.,-6.12323399573677E-17));
#5903=DIRECTION('center_axis',(-1.,0.,0.));
#5904=DIRECTION('ref_axis',(0.,-0.57126815541322,0.820763482746874));
#5905=DIRECTION('center_axis',(-1.,0.,0.));
#5906=DIRECTION('ref_axis',(0.,0.,1.));
#5907=DIRECTION('center_axis',(-1.,0.,0.));
#5908=DIRECTION('ref_axis',(0.,1.,0.));
#5909=DIRECTION('center_axis',(1.,0.,0.));
#5910=DIRECTION('ref_axis',(0.,-0.57126815541322,-0.820763482746874));
#5911=DIRECTION('center_axis',(1.,0.,0.));
#5912=DIRECTION('ref_axis',(0.,1.,0.));
#11788=CARTESIAN_POINT('',(0.,0.,0.));
#11789=CARTESIAN_POINT('Origin',(67.15,0.,0.));
#11790=CARTESIAN_POINT('',(67.3,12.6,-1.54305496692567E-15));
#11791=CARTESIAN_POINT('',(67.3,-12.6,-1.54305496692567E-15));
#11792=CARTESIAN_POINT('Origin',(67.3,0.,0.));
#11793=CARTESIAN_POINT('Origin',(67.3,0.,0.));
#11794=CARTESIAN_POINT('',(67.,12.3,1.50631556295124E-15));
#11795=CARTESIAN_POINT('',(67.15,12.45,1.52468526493846E-15));
#11796=CARTESIAN_POINT('Origin',(67.,0.,0.));
#11797=CARTESIAN_POINT('Origin',(67.6,0.,0.));
#11798=CARTESIAN_POINT('',(67.9,12.6,1.54305496692567E-15));
#11799=CARTESIAN_POINT('',(67.9,-12.6,-1.54305496692567E-15));
#11800=CARTESIAN_POINT('Origin',(67.9,0.,0.));
#11801=CARTESIAN_POINT('Origin',(67.9,0.,0.));
#11802=CARTESIAN_POINT('',(67.6,-12.6,-1.54305496692567E-15));
#11803=CARTESIAN_POINT('Origin',(67.,12.6,0.));
#11804=CARTESIAN_POINT('',(67.,-1.29812560709619E-15,10.6));
#11805=CARTESIAN_POINT('Origin',(67.,0.,0.));
#11806=CARTESIAN_POINT('Origin',(68.05,0.,0.));
#11807=CARTESIAN_POINT('',(68.2,12.3,-1.50631556295124E-15));
#11808=CARTESIAN_POINT('Origin',(68.2,0.,0.));
#11809=CARTESIAN_POINT('',(68.05,12.45,1.52468526493846E-15));
#11810=CARTESIAN_POINT('Origin',(68.2,10.5,0.));
#11811=CARTESIAN_POINT('',(68.2,-11.,-1.34711147906209E-15));
#11812=CARTESIAN_POINT('Origin',(68.2,0.,0.));
#11813=CARTESIAN_POINT('Origin',(67.6,0.,0.));
#11814=CARTESIAN_POINT('',(67.,10.24,-2.32215417231501));
#11815=CARTESIAN_POINT('',(68.2,10.24,-2.32215417231501));
#11816=CARTESIAN_POINT('',(67.6,10.24,-2.32215417231501));
#11817=CARTESIAN_POINT('',(67.,10.1980390271856,-2.5));
#11818=CARTESIAN_POINT('Origin',(67.,0.,0.));
#11819=CARTESIAN_POINT('',(68.2,10.1980390271856,-2.5));
#11820=CARTESIAN_POINT('',(67.6,10.1980390271856,-2.5));
#11821=CARTESIAN_POINT('Origin',(68.2,0.,0.));
#11822=CARTESIAN_POINT('Origin',(67.6,0.,0.));
#11823=CARTESIAN_POINT('',(68.2,10.24,2.32215417231501));
#11824=CARTESIAN_POINT('',(67.,10.24,2.32215417231501));
#11825=CARTESIAN_POINT('',(67.6,10.24,2.32215417231501));
#11826=CARTESIAN_POINT('',(68.2,10.1980390271856,2.5));
#11827=CARTESIAN_POINT('Origin',(68.2,0.,0.));
#11828=CARTESIAN_POINT('',(67.,10.1980390271856,2.5));
#11829=CARTESIAN_POINT('',(67.6,10.1980390271856,2.5));
#11830=CARTESIAN_POINT('Origin',(67.,0.,0.));
#11831=CARTESIAN_POINT('Origin',(68.2,10.5,0.));
#11832=CARTESIAN_POINT('',(68.2,10.24,-2.5));
#11833=CARTESIAN_POINT('',(68.2,10.24,0.));
#11834=CARTESIAN_POINT('',(68.2,9.56,-2.5));
#11835=CARTESIAN_POINT('Origin',(68.2,10.5,0.));
#11836=CARTESIAN_POINT('',(68.2,10.24,2.5));
#11837=CARTESIAN_POINT('',(68.2,10.24,0.));
#11838=CARTESIAN_POINT('',(68.2,9.56,2.5));
#11839=CARTESIAN_POINT('Origin',(67.,12.6,0.));
#11840=CARTESIAN_POINT('',(67.,10.24,-2.5));
#11841=CARTESIAN_POINT('',(67.,10.24,0.));
#11842=CARTESIAN_POINT('',(67.,10.61,-2.5));
#11843=CARTESIAN_POINT('Origin',(67.,12.6,0.));
#11844=CARTESIAN_POINT('',(67.,10.24,2.5));
#11845=CARTESIAN_POINT('',(67.,10.24,0.));
#11846=CARTESIAN_POINT('',(67.,10.61,2.5));
#11847=CARTESIAN_POINT('Origin',(58.5,8.62,2.5));
#11848=CARTESIAN_POINT('',(69.,10.24,2.5));
#11849=CARTESIAN_POINT('',(69.,10.24,2.5));
#11850=CARTESIAN_POINT('',(69.,7.9669630349337,2.5));
#11851=CARTESIAN_POINT('',(69.,7.,2.5));
#11852=CARTESIAN_POINT('',(69.0218379181362,7.83022988168291,2.5));
#11853=CARTESIAN_POINT('Ctrl Pts',(69.0218379181362,7.83022988168291,2.5));
#11854=CARTESIAN_POINT('Ctrl Pts',(69.0075947074924,7.87360329207051,2.5));
#11855=CARTESIAN_POINT('Ctrl Pts',(69.,7.92356314245502,2.5));
#11856=CARTESIAN_POINT('Ctrl Pts',(69.,7.96696303493369,2.5));
#11857=CARTESIAN_POINT('',(49.1,7.83022988168291,2.5));
#11858=CARTESIAN_POINT('',(59.6,7.83022988168291,2.5));
#11859=CARTESIAN_POINT('',(49.1000000000041,9.91907544765526,2.5));
#11860=CARTESIAN_POINT('',(49.1,9.56,2.5));
#11861=CARTESIAN_POINT('',(49.4711020394073,10.3051416724427,2.5));
#11862=CARTESIAN_POINT('Ctrl Pts',(49.471102006026,10.3051417027149,2.5));
#11863=CARTESIAN_POINT('Ctrl Pts',(49.3473096739212,10.176541099224,2.5));
#11864=CARTESIAN_POINT('Ctrl Pts',(49.2236056134068,10.0478555238674,2.5));
#11865=CARTESIAN_POINT('Ctrl Pts',(49.1000000000083,9.91907544765526,2.5));
#11866=CARTESIAN_POINT('',(49.2908747206533,10.7048947780346,2.50000000015575));
#11867=CARTESIAN_POINT('Ctrl Pts',(49.4711018427219,10.3051416733467,2.49999916236061));
#11868=CARTESIAN_POINT('Ctrl Pts',(49.4521138045415,10.3172467342247,2.4999991258175));
#11869=CARTESIAN_POINT('Ctrl Pts',(49.434143505605,10.330934192123,2.49999638873673));
#11870=CARTESIAN_POINT('Ctrl Pts',(49.4173733976671,10.3460508501851,2.49999630498322));
#11871=CARTESIAN_POINT('Ctrl Pts',(49.4122331919494,10.3506842569879,2.49999627931193));
#11872=CARTESIAN_POINT('Ctrl Pts',(49.407206024932,10.3554521608227,2.49999644341522));
#11873=CARTESIAN_POINT('Ctrl Pts',(49.4022979734507,10.3603506775391,2.49999677600973));
#11874=CARTESIAN_POINT('Ctrl Pts',(49.3864116942846,10.3762060947765,2.49999785254475));
#11875=CARTESIAN_POINT('Ctrl Pts',(49.3718997498427,10.39329834119,2.50000118698146));
#11876=CARTESIAN_POINT('Ctrl Pts',(49.3589269316826,10.4114566220581,2.50000300029283));
#11877=CARTESIAN_POINT('Ctrl Pts',(49.350246313729,10.4236070350959,2.5000042136501));
#11878=CARTESIAN_POINT('Ctrl Pts',(49.3422554681063,10.4362356041593,2.50000459747335));
#11879=CARTESIAN_POINT('Ctrl Pts',(49.3350146148726,10.4492980430834,2.50000044385569));
#11880=CARTESIAN_POINT('Ctrl Pts',(49.3281858085234,10.4616171528597,2.49999652660315));
#11881=CARTESIAN_POINT('Ctrl Pts',(49.322024170055,10.4743223572284,2.49998855549731));
#11882=CARTESIAN_POINT('Ctrl Pts',(49.3165487906394,10.4873606414204,2.49998021758341));
#11883=CARTESIAN_POINT('Ctrl Pts',(49.3078883482859,10.5079833782326,2.49996702945212));
#11884=CARTESIAN_POINT('Ctrl Pts',(49.3010202713955,10.5292527079667,2.49995372503714));
#11885=CARTESIAN_POINT('Ctrl Pts',(49.295964487035,10.5509344138267,2.49994954600057));
#11886=CARTESIAN_POINT('Ctrl Pts',(49.2909278369453,10.5725340624628,2.49994538278011));
#11887=CARTESIAN_POINT('Ctrl Pts',(49.2876895556668,10.5945443716744,2.49995033506508));
#11888=CARTESIAN_POINT('Ctrl Pts',(49.2863171078659,10.616744070017,2.49996099739857));
#11889=CARTESIAN_POINT('Ctrl Pts',(49.2859316121374,10.6229795631829,2.49996399225492));
#11890=CARTESIAN_POINT('Ctrl Pts',(49.2856936230256,10.6292299902788,2.49996735822794));
#11891=CARTESIAN_POINT('Ctrl Pts',(49.2856053589302,10.6354903616755,2.49997082976491));
#11892=CARTESIAN_POINT('Ctrl Pts',(49.2852767142312,10.6588003821638,2.49998375577085));
#11893=CARTESIAN_POINT('Ctrl Pts',(49.2870227193347,10.6820201214405,2.49999973692703));
#11894=CARTESIAN_POINT('Ctrl Pts',(49.2908747205558,10.7048947773733,2.49999999901159));
#11895=CARTESIAN_POINT('',(49.3656854249492,10.7121426428143,2.5));
#11896=CARTESIAN_POINT('Ctrl Pts',(49.3656854249492,10.7121426428143,2.5));
#11897=CARTESIAN_POINT('Ctrl Pts',(49.3420008434391,10.7121426428143,2.5));
#11898=CARTESIAN_POINT('Ctrl Pts',(49.316211839325,10.7098484152381,2.5));
#11899=CARTESIAN_POINT('Ctrl Pts',(49.2908747205092,10.7048947787715,2.5));
#11900=CARTESIAN_POINT('',(50.0760927660041,10.7121954410373,2.49981008259284));
#11901=CARTESIAN_POINT('',(58.1,10.7121426428143,2.5));
#11902=CARTESIAN_POINT('',(50.4873080527574,10.24,2.5000000001691));
#11903=CARTESIAN_POINT('Ctrl Pts',(50.0760927937211,10.7121954053708,2.49981021088675));
#11904=CARTESIAN_POINT('Ctrl Pts',(50.0724347185981,10.6931913800779,2.49980703933385));
#11905=CARTESIAN_POINT('Ctrl Pts',(50.0702493871277,10.6739403201419,2.4997968810974));
#11906=CARTESIAN_POINT('Ctrl Pts',(50.069525629523,10.654595400641,2.49979096643753));
#11907=CARTESIAN_POINT('Ctrl Pts',(50.0687949509244,10.6350654936968,2.49978499521822));
#11908=CARTESIAN_POINT('Ctrl Pts',(50.0695567922128,10.6155130900928,2.49978334870012));
#11909=CARTESIAN_POINT('Ctrl Pts',(50.0717964790934,10.5960964549971,2.49978810400288));
#11910=CARTESIAN_POINT('Ctrl Pts',(50.074056422491,10.576504209014,2.49979290231427));
#11911=CARTESIAN_POINT('Ctrl Pts',(50.0778126805385,10.5571242161645,2.49980421827627));
#11912=CARTESIAN_POINT('Ctrl Pts',(50.0830446502572,10.5381168834534,2.49981480884476));
#11913=CARTESIAN_POINT('Ctrl Pts',(50.085301988002,10.5299161537353,2.49981937815446));
#11914=CARTESIAN_POINT('Ctrl Pts',(50.0878292904794,10.5218034036804,2.49982375513529));
#11915=CARTESIAN_POINT('Ctrl Pts',(50.0906226140567,10.5137908789098,2.49982683752301));
#11916=CARTESIAN_POINT('Ctrl Pts',(50.0979560533961,10.4927552334733,2.49983492985557));
#11917=CARTESIAN_POINT('Ctrl Pts',(50.1071191248528,10.4724097745267,2.49983508259961));
#11918=CARTESIAN_POINT('Ctrl Pts',(50.1179434009193,10.4529284325733,2.49984014939377));
#11919=CARTESIAN_POINT('Ctrl Pts',(50.1223596888886,10.4449800750514,2.49984221663798));
#11920=CARTESIAN_POINT('Ctrl Pts',(50.1270531075935,10.4371756491499,2.49984495292356));
#11921=CARTESIAN_POINT('Ctrl Pts',(50.1320145050724,10.4295276315651,2.49984866910354));
#11922=CARTESIAN_POINT('Ctrl Pts',(50.1445994971712,10.4101278069619,2.4998580954992));
#11923=CARTESIAN_POINT('Ctrl Pts',(50.1588049548903,10.3918873519457,2.49987278486773));
#11924=CARTESIAN_POINT('Ctrl Pts',(50.1744316650975,10.374977827846,2.49989012485888));
#11925=CARTESIAN_POINT('Ctrl Pts',(50.1841474977131,10.3644644118048,2.49990090591576));
#11926=CARTESIAN_POINT('Ctrl Pts',(50.1944138546499,10.3544654862454,2.49991239300784));
#11927=CARTESIAN_POINT('Ctrl Pts',(50.2051921016056,10.345025159572,2.49992124592571));
#11928=CARTESIAN_POINT('Ctrl Pts',(50.2160584446486,10.3355076723135,2.49993017120298));
#11929=CARTESIAN_POINT('Ctrl Pts',(50.2274450835419,10.326557775575,2.49993643693284));
#11930=CARTESIAN_POINT('Ctrl Pts',(50.2392963798676,10.3182015287255,2.49994151742415));
#11931=CARTESIAN_POINT('Ctrl Pts',(50.2582120637921,10.3048642430937,2.4999496263234));
#11932=CARTESIAN_POINT('Ctrl Pts',(50.2781856685745,10.2931249989061,2.49995479742236));
#11933=CARTESIAN_POINT('Ctrl Pts',(50.2989721259798,10.2830646910121,2.49996241168663));
#11934=CARTESIAN_POINT('Ctrl Pts',(50.3116765962231,10.2769159336849,2.49996706544709));
#11935=CARTESIAN_POINT('Ctrl Pts',(50.3246856114912,10.2713948751988,2.49997229683092));
#11936=CARTESIAN_POINT('Ctrl Pts',(50.3379495491142,10.2665266123185,2.49997672454703));
#11937=CARTESIAN_POINT('Ctrl Pts',(50.3446721543995,10.2640592145743,2.499978968661));
#11938=CARTESIAN_POINT('Ctrl Pts',(50.3514603069851,10.2617595967717,2.49998097829715));
#11939=CARTESIAN_POINT('Ctrl Pts',(50.3583070707371,10.2596289619541,2.49998265182534));
#11940=CARTESIAN_POINT('Ctrl Pts',(50.3807108950684,10.2526571472551,2.49998812790615));
#11941=CARTESIAN_POINT('Ctrl Pts',(50.4036318885686,10.2475250346903,2.49999069009023));
#11942=CARTESIAN_POINT('Ctrl Pts',(50.4268185719221,10.244255753949,2.49999402764095));
#11943=CARTESIAN_POINT('Ctrl Pts',(50.4468344518825,10.2414335507957,2.49999690877808));
#11944=CARTESIAN_POINT('Ctrl Pts',(50.4670493379255,10.24,2.49999999999998));
#11945=CARTESIAN_POINT('Ctrl Pts',(50.4873080526582,10.24,2.5));
#11946=CARTESIAN_POINT('',(69.,10.24,2.5));
#11947=CARTESIAN_POINT('Ctrl Pts',(50.10596357807,10.6854183957887,2.61186402918292));
#11948=CARTESIAN_POINT('Ctrl Pts',(50.0460788562875,10.7408164456412,2.38522461213428));
#11949=CARTESIAN_POINT('Ctrl Pts',(49.9164083980935,10.8391161748358,1.92156092596857));
#11950=CARTESIAN_POINT('Ctrl Pts',(49.7576509378753,10.9271110146993,1.30914434152331));
#11951=CARTESIAN_POINT('Ctrl Pts',(49.666672528926,10.967422685746,0.865348982805604));
#11952=CARTESIAN_POINT('Ctrl Pts',(49.6243567523392,10.9841733422946,0.604311373359717));
#11953=CARTESIAN_POINT('Ctrl Pts',(49.5997258546835,10.9933200965768,0.404693900681247));
#11954=CARTESIAN_POINT('Ctrl Pts',(49.5716547215071,11.0027241723402,0.0691641331704865));
#11955=CARTESIAN_POINT('Ctrl Pts',(49.5900774295882,10.9974150814697,-0.476621441399214));
#11956=CARTESIAN_POINT('Ctrl Pts',(49.7280572779163,10.9444131408942,-1.18870751171882));
#11957=CARTESIAN_POINT('Ctrl Pts',(49.915841181391,10.8391437000355,-1.92085485622915));
#11958=CARTESIAN_POINT('Ctrl Pts',(50.0460661791746,10.7408281729562,-2.38517663440393));
#11959=CARTESIAN_POINT('Ctrl Pts',(50.1059635780249,10.6854183958305,-2.61186402901213));
#11960=CARTESIAN_POINT('Ctrl Pts',(50.0989714172686,10.6216586600213,2.6139151177149));
#11961=CARTESIAN_POINT('Ctrl Pts',(50.0300443077418,10.672816415315,2.39024416325827));
#11962=CARTESIAN_POINT('Ctrl Pts',(49.8808171508488,10.7675718810144,1.93499669767664));
#11963=CARTESIAN_POINT('Ctrl Pts',(49.6975309544909,10.862958211197,1.33199623935741));
#11964=CARTESIAN_POINT('Ctrl Pts',(49.5912646760291,10.912041457587,0.888629458300868));
#11965=CARTESIAN_POINT('Ctrl Pts',(49.5411396412093,10.9338315137794,0.624351882943105));
#11966=CARTESIAN_POINT('Ctrl Pts',(49.5117069919845,10.9462019721493,0.420209333159837));
#11967=CARTESIAN_POINT('Ctrl Pts',(49.4773242232257,10.9598077704949,0.0728776092390634));
#11968=CARTESIAN_POINT('Ctrl Pts',(49.5006330977212,10.9512789811939,-0.498940433437269));
#11969=CARTESIAN_POINT('Ctrl Pts',(49.6638979089462,10.8811822008758,-1.21335763832631));
#11970=CARTESIAN_POINT('Ctrl Pts',(49.8800144260071,10.7677624922463,-1.93434775525291));
#11971=CARTESIAN_POINT('Ctrl Pts',(50.0300297164284,10.6728272449952,-2.39019681392804));
#11972=CARTESIAN_POINT('Ctrl Pts',(50.0989714172167,10.6216586600599,-2.61391511754634));
#11973=CARTESIAN_POINT('Ctrl Pts',(50.1150024369948,10.4905936402599,2.60921255985761));
#11974=CARTESIAN_POINT('Ctrl Pts',(50.0322851458687,10.5282606753826,2.3888654393634));
#11975=CARTESIAN_POINT('Ctrl Pts',(49.8507006451456,10.602551600071,1.94594986862127));
#11976=CARTESIAN_POINT('Ctrl Pts',(49.6201589477057,10.6899004066302,1.36161040345567));
#11977=CARTESIAN_POINT('Ctrl Pts',(49.4811686636315,10.7412549980383,0.922685634553976));
#11978=CARTESIAN_POINT('Ctrl Pts',(49.4137309602737,10.7655984033572,0.655012650144937));
#11979=CARTESIAN_POINT('Ctrl Pts',(49.3734928710052,10.7799234763981,0.444625304668301));
#11980=CARTESIAN_POINT('Ctrl Pts',(49.3247495826024,10.796604039827,0.0790162780648425));
#11981=CARTESIAN_POINT('Ctrl Pts',(49.3592937415449,10.7853242476646,-0.535131696197622));
#11982=CARTESIAN_POINT('Ctrl Pts',(49.5791556288816,10.7058491105962,-1.24644054242593));
#11983=CARTESIAN_POINT('Ctrl Pts',(49.8493254724924,10.60293912814,-1.94543141854448));
#11984=CARTESIAN_POINT('Ctrl Pts',(50.0322676352843,10.5282686491883,-2.38881879366335));
#11985=CARTESIAN_POINT('Ctrl Pts',(50.1150024369325,10.4905936402883,-2.60921255969157));
#11986=CARTESIAN_POINT('Ctrl Pts',(50.2146309334458,10.3415545946635,2.57998742154472));
#11987=CARTESIAN_POINT('Ctrl Pts',(50.1280147436699,10.3579163649357,2.35632872799266));
#11988=CARTESIAN_POINT('Ctrl Pts',(49.9329267878874,10.3913302277352,1.91381270831632));
#11989=CARTESIAN_POINT('Ctrl Pts',(49.6753913671128,10.4341807413213,1.34149299628219));
#11990=CARTESIAN_POINT('Ctrl Pts',(49.515517131939,10.4611489433235,0.912449575184171));
#11991=CARTESIAN_POINT('Ctrl Pts',(49.4368991664712,10.4743372237122,0.649532628539433));
#11992=CARTESIAN_POINT('Ctrl Pts',(49.3896820250642,10.4822188796987,0.441974264929375));
#11993=CARTESIAN_POINT('Ctrl Pts',(49.331903164895,10.4916293139201,0.0790634742199547));
#11994=CARTESIAN_POINT('Ctrl Pts',(49.3733374267131,10.4850633550494,-0.53401775304525));
#11995=CARTESIAN_POINT('Ctrl Pts',(49.6302127509665,10.441780875437,-1.22860722352935));
#11996=CARTESIAN_POINT('Ctrl Pts',(49.931195998432,10.3915871925538,-1.91338712054486));
#11997=CARTESIAN_POINT('Ctrl Pts',(50.1279964077188,10.35791982859,-2.35628138126123));
#11998=CARTESIAN_POINT('Ctrl Pts',(50.2146309333805,10.3415545946759,-2.57998742137617));
#11999=CARTESIAN_POINT('Ctrl Pts',(50.3487993253124,10.2576120585743,2.54063031038476));
#12000=CARTESIAN_POINT('Ctrl Pts',(50.268468199078,10.2605598936513,2.30911926875332));
#12001=CARTESIAN_POINT('Ctrl Pts',(50.0829097045463,10.2667082145781,1.85595146364309));
#12002=CARTESIAN_POINT('Ctrl Pts',(49.834412994289,10.2748729796263,1.28196538532196));
#12003=CARTESIAN_POINT('Ctrl Pts',(49.680835270301,10.280139448227,0.861728214240658));
#12004=CARTESIAN_POINT('Ctrl Pts',(49.6060998009801,10.2827398747948,0.608877935796896));
#12005=CARTESIAN_POINT('Ctrl Pts',(49.5614948221163,10.2843033157519,0.411842146135796));
#12006=CARTESIAN_POINT('Ctrl Pts',(49.5079282298224,10.286183251424,0.0724642239699666));
#12007=CARTESIAN_POINT('Ctrl Pts',(49.5454900245608,10.2848624181149,-0.49295565087574));
#12008=CARTESIAN_POINT('Ctrl Pts',(49.7901458075476,10.2763008155086,-1.1689093490474));
#12009=CARTESIAN_POINT('Ctrl Pts',(50.0814081572479,10.2667616581884,-1.85544105748007));
#12010=CARTESIAN_POINT('Ctrl Pts',(50.2684511936231,10.2605605176842,-2.30907025974476));
#12011=CARTESIAN_POINT('Ctrl Pts',(50.3487993252519,10.2576120585765,-2.5406303102103));
#12012=CARTESIAN_POINT('Ctrl Pts',(50.4411230608376,10.24,2.51354795908566));
#12013=CARTESIAN_POINT('Ctrl Pts',(50.3672699512713,10.2399851855682,2.27600839076339));
#12014=CARTESIAN_POINT('Ctrl Pts',(50.1936849991744,10.2399659210815,1.81340446242885));
#12015=CARTESIAN_POINT('Ctrl Pts',(49.9605600409879,10.2399459207391,1.2347012119753));
#12016=CARTESIAN_POINT('Ctrl Pts',(49.8184924102703,10.2399466460418,0.819505327343819));
#12017=CARTESIAN_POINT('Ctrl Pts',(49.7504193447077,10.2399497034154,0.574248649565897));
#12018=CARTESIAN_POINT('Ctrl Pts',(49.7101658107336,10.2399531561777,0.385760776646267));
#12019=CARTESIAN_POINT('Ctrl Pts',(49.6629992153512,10.2399589729157,0.0665545800454013));
#12020=CARTESIAN_POINT('Ctrl Pts',(49.6950815292353,10.239953993875,-0.456754223466842));
#12021=CARTESIAN_POINT('Ctrl Pts',(49.9181644279458,10.239937833965,-1.12092692435959));
#12022=CARTESIAN_POINT('Ctrl Pts',(50.1924973076596,10.2399668152967,-1.81280733835446));
#12023=CARTESIAN_POINT('Ctrl Pts',(50.3672543171596,10.2399851824321,-2.27595810556525));
#12024=CARTESIAN_POINT('Ctrl Pts',(50.441123060782,10.24,-2.51354795890666));
#12025=CARTESIAN_POINT('Ctrl Pts',(50.4873080527118,10.24,2.5000000001825));
#12026=CARTESIAN_POINT('Ctrl Pts',(50.4167383525177,10.24,2.25942789236011));
#12027=CARTESIAN_POINT('Ctrl Pts',(50.2491743046301,10.24,1.79205452172678));
#12028=CARTESIAN_POINT('Ctrl Pts',(50.0239314790447,10.24,1.21089457224777));
#12029=CARTESIAN_POINT('Ctrl Pts',(49.8878049235054,10.24,0.798190480225308));
#12030=CARTESIAN_POINT('Ctrl Pts',(49.8231790425819,10.24,0.556751291784615));
#12031=CARTESIAN_POINT('Ctrl Pts',(49.7851714883371,10.24,0.372575689154406));
#12032=CARTESIAN_POINT('Ctrl Pts',(49.7413090623653,10.24,0.0635723530955229));
#12033=CARTESIAN_POINT('Ctrl Pts',(49.7705555891009,10.24,-0.43840113636878));
#12034=CARTESIAN_POINT('Ctrl Pts',(49.9825087104814,10.24,-1.09672361261615));
#12035=CARTESIAN_POINT('Ctrl Pts',(50.2481483914462,10.24,-1.79140201558762));
#12036=CARTESIAN_POINT('Ctrl Pts',(50.4167234134771,10.24,-2.25937696519828));
#12037=CARTESIAN_POINT('Ctrl Pts',(50.4873080526586,10.24,-2.50000000000121));
#12038=CARTESIAN_POINT('',(50.4873080526589,10.24,-2.50000000000112));
#12039=CARTESIAN_POINT('',(50.0760766664832,10.712193812233,-2.49979592332684));
#12040=CARTESIAN_POINT('Ctrl Pts',(50.4873080526582,10.24,-2.5));
#12041=CARTESIAN_POINT('Ctrl Pts',(50.4641571594583,10.24,-2.5));
#12042=CARTESIAN_POINT('Ctrl Pts',(50.4410809471426,10.2418709746727,-2.49999428716151));
#12043=CARTESIAN_POINT('Ctrl Pts',(50.4183088007534,10.2455410414974,-2.49998945021977));
#12044=CARTESIAN_POINT('Ctrl Pts',(50.3953275608783,10.2492448068172,-2.49998456886531));
#12045=CARTESIAN_POINT('Ctrl Pts',(50.3726546190859,10.2547813030666,-2.49998094173844));
#12046=CARTESIAN_POINT('Ctrl Pts',(50.3505360224068,10.2621263928632,-2.4999763370001));
#12047=CARTESIAN_POINT('Ctrl Pts',(50.3463173584445,10.2635273165327,-2.49997545874168));
#12048=CARTESIAN_POINT('Ctrl Pts',(50.3421189250459,10.2649941656051,-2.49997450960908));
#12049=CARTESIAN_POINT('Ctrl Pts',(50.3379425354016,10.2665269556365,-2.499973420438));
#12050=CARTESIAN_POINT('Ctrl Pts',(50.3319465679701,10.2687275546922,-2.49997185673468));
#12051=CARTESIAN_POINT('Ctrl Pts',(50.3259960277548,10.2710640639799,-2.49997000822049));
#12052=CARTESIAN_POINT('Ctrl Pts',(50.3200958828164,10.2735348019973,-2.49996776320823));
#12053=CARTESIAN_POINT('Ctrl Pts',(50.2989516264854,10.2823891468498,-2.49995971779324));
#12054=CARTESIAN_POINT('Ctrl Pts',(50.2785893166508,10.2929069318771,-2.49994874716809));
#12055=CARTESIAN_POINT('Ctrl Pts',(50.2592178604724,10.3049773058068,-2.4999397329224));
#12056=CARTESIAN_POINT('Ctrl Pts',(50.2401649112326,10.316849217741,-2.49993086688961));
#12057=CARTESIAN_POINT('Ctrl Pts',(50.222069498692,10.3302239956641,-2.49992413432698));
#12058=CARTESIAN_POINT('Ctrl Pts',(50.2051646417189,10.3450289994691,-2.49991117822164));
#12059=CARTESIAN_POINT('Ctrl Pts',(50.197210595605,10.3519950260477,-2.4999050821358));
#12060=CARTESIAN_POINT('Ctrl Pts',(50.1895207594136,10.3592781180278,-2.49989737920897));
#12061=CARTESIAN_POINT('Ctrl Pts',(50.1821140026648,10.3668627737153,-2.49988876547526));
#12062=CARTESIAN_POINT('Ctrl Pts',(50.165999922145,10.3833638897375,-2.49987002550536));
#12063=CARTESIAN_POINT('Ctrl Pts',(50.151356493375,10.4011543565194,-2.49985067555682));
#12064=CARTESIAN_POINT('Ctrl Pts',(50.1383299981319,10.4200373670364,-2.49983801584716));
#12065=CARTESIAN_POINT('Ctrl Pts',(50.1257967192861,10.4382054185223,-2.49982583546645));
#12066=CARTESIAN_POINT('Ctrl Pts',(50.1147597288176,10.4573861991229,-2.49981998122588));
#12067=CARTESIAN_POINT('Ctrl Pts',(50.105392687849,10.4774188980176,-2.49981541575245));
#12068=CARTESIAN_POINT('Ctrl Pts',(50.1021188952813,10.4844203514085,-2.49981382011376));
#12069=CARTESIAN_POINT('Ctrl Pts',(50.0990495236464,10.4915259093987,-2.4998122667488));
#12070=CARTESIAN_POINT('Ctrl Pts',(50.096193480471,10.4987286999449,-2.49981014733828));
#12071=CARTESIAN_POINT('Ctrl Pts',(50.0942154074463,10.5037172959875,-2.49980867945124));
#12072=CARTESIAN_POINT('Ctrl Pts',(50.0923436965187,10.5087424589632,-2.49980700430729));
#12073=CARTESIAN_POINT('Ctrl Pts',(50.090580189988,10.5138015741308,-2.49980482970845));
#12074=CARTESIAN_POINT('Ctrl Pts',(50.0830548124857,10.535390238988,-2.49979555008463));
#12075=CARTESIAN_POINT('Ctrl Pts',(50.0774959148627,10.557596686582,-2.49977795996577));
#12076=CARTESIAN_POINT('Ctrl Pts',(50.0739341814136,10.5801728194331,-2.49976761437599));
#12077=CARTESIAN_POINT('Ctrl Pts',(50.0726394342436,10.5883796054086,-2.49976385358836));
#12078=CARTESIAN_POINT('Ctrl Pts',(50.0716090801445,10.5966352786126,-2.49976095198664));
#12079=CARTESIAN_POINT('Ctrl Pts',(50.0708462864984,10.604927788451,-2.4997593080838));
#12080=CARTESIAN_POINT('Ctrl Pts',(50.0688248378512,10.6269034340006,-2.49975495164327));
#12081=CARTESIAN_POINT('Ctrl Pts',(50.0686944970557,10.6489677176883,-2.49976023269914));
#12082=CARTESIAN_POINT('Ctrl Pts',(50.0704571109796,10.6708939952819,-2.49976785447707));
#12083=CARTESIAN_POINT('Ctrl Pts',(50.0715698352885,10.6847358818991,-2.49977266604554));
#12084=CARTESIAN_POINT('Ctrl Pts',(50.0734379057857,10.6985230156386,-2.49977821610713));
#12085=CARTESIAN_POINT('Ctrl Pts',(50.0760723344211,10.7121976923269,-2.49978044852387));
#12086=CARTESIAN_POINT('Ctrl Pts',(50.4873080526586,10.24,-2.50000000000121));
#12087=CARTESIAN_POINT('Ctrl Pts',(50.4167234134771,10.24,-2.25937696519828));
#12088=CARTESIAN_POINT('Ctrl Pts',(50.2481483914462,10.24,-1.79140201558762));
#12089=CARTESIAN_POINT('Ctrl Pts',(49.9825087104814,10.24,-1.09672361261615));
#12090=CARTESIAN_POINT('Ctrl Pts',(49.7705555891009,10.24,-0.43840113636878));
#12091=CARTESIAN_POINT('Ctrl Pts',(49.7413090623653,10.24,0.0635723530955229));
#12092=CARTESIAN_POINT('Ctrl Pts',(49.7851714883371,10.24,0.372575689154406));
#12093=CARTESIAN_POINT('Ctrl Pts',(49.8231790425819,10.24,0.556751291784615));
#12094=CARTESIAN_POINT('Ctrl Pts',(49.8878049235054,10.24,0.798190480225308));
#12095=CARTESIAN_POINT('Ctrl Pts',(50.0239314790447,10.24,1.21089457224777));
#12096=CARTESIAN_POINT('Ctrl Pts',(50.2491743046301,10.24,1.79205452172678));
#12097=CARTESIAN_POINT('Ctrl Pts',(50.4167383525177,10.24,2.25942789236011));
#12098=CARTESIAN_POINT('Ctrl Pts',(50.4873080527118,10.24,2.5000000001825));
#12099=CARTESIAN_POINT('Ctrl Pts',(50.0760927937211,10.7121954053708,2.49981021088675));
#12100=CARTESIAN_POINT('Ctrl Pts',(50.0248077296735,10.7567670989664,2.30892405297712));
#12101=CARTESIAN_POINT('Ctrl Pts',(49.9707084492665,10.796890351521,2.11425277588037));
#12102=CARTESIAN_POINT('Ctrl Pts',(49.9170745205984,10.8321402105099,1.91499353062095));
#12103=CARTESIAN_POINT('Ctrl Pts',(49.8529054140062,10.8743141107812,1.67659429219047));
#12104=CARTESIAN_POINT('Ctrl Pts',(49.7894024299189,10.9095120467266,1.43162765841236));
#12105=CARTESIAN_POINT('Ctrl Pts',(49.733576327052,10.9366015191072,1.18090721526053));
#12106=CARTESIAN_POINT('Ctrl Pts',(49.7056632756186,10.9501462552974,1.05554699368462));
#12107=CARTESIAN_POINT('Ctrl Pts',(49.6796694444902,10.9616638755964,0.928748319765275));
#12108=CARTESIAN_POINT('Ctrl Pts',(49.6568995752518,10.9710866345457,0.799469558643532));
#12109=CARTESIAN_POINT('Ctrl Pts',(49.6455146406326,10.9757980140203,0.73483017808266));
#12110=CARTESIAN_POINT('Ctrl Pts',(49.6349356964859,10.9799856781574,0.669570775721189));
#12111=CARTESIAN_POINT('Ctrl Pts',(49.6255410748033,10.983603969273,0.603671495760708));
#12112=CARTESIAN_POINT('Ctrl Pts',(49.6161464531206,10.9872222603887,0.537772215800227));
#12113=CARTESIAN_POINT('Ctrl Pts',(49.6079361539021,10.9902711784827,0.471233058240737));
#12114=CARTESIAN_POINT('Ctrl Pts',(49.6010238909752,10.9927360451061,0.404410502709916));
#12115=CARTESIAN_POINT('Ctrl Pts',(49.5941116280482,10.9952009117295,0.337587947179095));
#12116=CARTESIAN_POINT('Ctrl Pts',(49.5884974014129,10.9970817268822,0.270481993676943));
#12117=CARTESIAN_POINT('Ctrl Pts',(49.584862441064,10.998326429157,0.203096729345026));
#12118=CARTESIAN_POINT('Ctrl Pts',(49.5739575600172,11.0020605359813,0.000940936349274404));
#12119=CARTESIAN_POINT('Ctrl Pts',(49.5808660755476,11.0000696269049,-0.203728654114363));
#12120=CARTESIAN_POINT('Ctrl Pts',(49.6009413134475,10.9927369325602,-0.403913545195877));
#12121=CARTESIAN_POINT('Ctrl Pts',(49.6277082973141,10.9829600067673,-0.670826733304562));
#12122=CARTESIAN_POINT('Ctrl Pts',(49.6778827876152,10.9636865738307,-0.929767122511692));
#12123=CARTESIAN_POINT('Ctrl Pts',(49.7342673500115,10.9365049505527,-1.18126187453365));
#12124=CARTESIAN_POINT('Ctrl Pts',(49.7906519124079,10.9093233272746,-1.4327566265556));
#12125=CARTESIAN_POINT('Ctrl Pts',(49.8532465468994,10.8742335136551,-1.67680574139238));
#12126=CARTESIAN_POINT('Ctrl Pts',(49.9171001135911,10.8321097250754,-1.91491074335446));
#12127=CARTESIAN_POINT('Ctrl Pts',(49.9704714803631,10.7969009765812,-2.1139284341172));
#12128=CARTESIAN_POINT('Ctrl Pts',(50.0247223731089,10.7567780923798,-2.30879339793801));
#12129=CARTESIAN_POINT('Ctrl Pts',(50.0760723344211,10.7121976923269,-2.49978044852387));
#12130=CARTESIAN_POINT('Origin',(69.8343145750508,0.,0.));
#12131=CARTESIAN_POINT('',(70.1171572875254,-1.33276384934561E-15,10.8828427124746));
#12132=CARTESIAN_POINT('',(70.1171572875254,-10.8828427124746,-1.33276384934562E-15));
#12133=CARTESIAN_POINT('Origin',(70.1171572875254,0.,-1.66595481168202E-15));
#12134=CARTESIAN_POINT('Origin',(70.1171572875254,0.,-1.66595481168202E-15));
#12135=CARTESIAN_POINT('',(69.8343145750508,-1.34711147906209E-15,11.));
#12136=CARTESIAN_POINT('Origin',(69.8343145750508,-1.29812560709619E-15,
10.6));
#12137=CARTESIAN_POINT('',(69.8343145750508,-11.,-1.34711147906209E-15));
#12138=CARTESIAN_POINT('Origin',(69.8343145750508,0.,0.));
#12139=CARTESIAN_POINT('Origin',(69.8343145750508,0.,0.));
#12140=CARTESIAN_POINT('Origin',(68.9,0.,0.));
#12141=CARTESIAN_POINT('',(68.9,-11.,-1.34711147906209E-15));
#12142=CARTESIAN_POINT('Origin',(70.25,0.,0.));
#12143=CARTESIAN_POINT('',(70.3828427124746,-10.6171572875254,-1.3002267688212E-15));
#12144=CARTESIAN_POINT('',(70.3828427124746,-1.3002267688212E-15,10.6171572875254));
#12145=CARTESIAN_POINT('Origin',(70.3828427124746,0.,-1.62528346102649E-15));
#12146=CARTESIAN_POINT('',(70.25,-10.75,-1.3164953090834E-15));
#12147=CARTESIAN_POINT('Origin',(70.3828427124746,0.,-1.62528346102649E-15));
#12148=CARTESIAN_POINT('Origin',(66.6,0.,0.));
#12149=CARTESIAN_POINT('',(66.6,-1.34711147906209E-15,11.));
#12150=CARTESIAN_POINT('Origin',(66.6,-1.29812560709619E-15,10.6));
#12151=CARTESIAN_POINT('',(66.6,-11.,-1.34711147906209E-15));
#12152=CARTESIAN_POINT('Origin',(66.6,0.,0.));
#12153=CARTESIAN_POINT('Origin',(66.6,0.,0.));
#12154=CARTESIAN_POINT('Origin',(58.1,0.,0.));
#12155=CARTESIAN_POINT('',(49.3656854249492,-11.,-1.34711147906209E-15));
#12156=CARTESIAN_POINT('',(58.1,-11.,-1.34711147906209E-15));
#12157=CARTESIAN_POINT('',(49.3656854249492,10.7121426428143,-2.5));
#12158=CARTESIAN_POINT('Origin',(49.3656854249492,0.,0.));
#12159=CARTESIAN_POINT('',(58.1,10.7121426428143,-2.5));
#12160=CARTESIAN_POINT('Origin',(49.3656854249492,0.,0.));
#12161=CARTESIAN_POINT('Origin',(49.3656854249492,0.,0.));
#12162=CARTESIAN_POINT('',(49.290874720642,10.7048947780099,-2.50000000016032));
#12163=CARTESIAN_POINT('Ctrl Pts',(49.2908747204936,10.7048947787685,-2.5));
#12164=CARTESIAN_POINT('Ctrl Pts',(49.3162118393145,10.7098484152371,-2.5));
#12165=CARTESIAN_POINT('Ctrl Pts',(49.3420008434342,10.7121426428143,-2.5));
#12166=CARTESIAN_POINT('Ctrl Pts',(49.3656854249492,10.7121426428143,-2.5));
#12167=CARTESIAN_POINT('',(49.3323331704973,10.6616743509686,2.70149187398907));
#12168=CARTESIAN_POINT('Ctrl Pts',(49.2908747206827,10.7048947779969,2.4999999991104));
#12169=CARTESIAN_POINT('Ctrl Pts',(49.3045010041015,10.6906254142154,2.5724257382579));
#12170=CARTESIAN_POINT('Ctrl Pts',(49.3184413442248,10.6761441724483,2.63964675585704));
#12171=CARTESIAN_POINT('Ctrl Pts',(49.3323950806311,10.6616812501835,2.70147713019892));
#12172=CARTESIAN_POINT('',(49.0828426943265,10.4676389273726,2.97738149942411));
#12173=CARTESIAN_POINT('Ctrl Pts',(49.3324087881176,10.6616015016905,2.70162046046199));
#12174=CARTESIAN_POINT('Ctrl Pts',(49.3135649567906,10.6557614583055,2.71827621407867));
#12175=CARTESIAN_POINT('Ctrl Pts',(49.2952674330737,10.6484809566042,2.73524347292328));
#12176=CARTESIAN_POINT('Ctrl Pts',(49.2776083070661,10.6399566490912,2.75232179660182));
#12177=CARTESIAN_POINT('Ctrl Pts',(49.2689844692774,10.6357938017781,2.76066199945467));
#12178=CARTESIAN_POINT('Ctrl Pts',(49.2605129098377,10.6313342979202,2.76902953786562));
#12179=CARTESIAN_POINT('Ctrl Pts',(49.2522046371122,10.626600777531,2.77740545786278));
#12180=CARTESIAN_POINT('Ctrl Pts',(49.2346176799969,10.6165808584889,2.79513561076665));
#12181=CARTESIAN_POINT('Ctrl Pts',(49.217760859958,10.6053345841082,2.81290035916848));
#12182=CARTESIAN_POINT('Ctrl Pts',(49.2016912137775,10.5931223499357,2.83054337312961));
#12183=CARTESIAN_POINT('Ctrl Pts',(49.199028540575,10.5910988337793,2.83346674679688));
#12184=CARTESIAN_POINT('Ctrl Pts',(49.1963875221415,10.5890487558497,2.83638687761696));
#12185=CARTESIAN_POINT('Ctrl Pts',(49.1937684684831,10.5869732520537,2.83930316752249));
#12186=CARTESIAN_POINT('Ctrl Pts',(49.1749952468881,10.5720961636983,2.86020696094277));
#12187=CARTESIAN_POINT('Ctrl Pts',(49.1571526657491,10.5557556236773,2.88110859508633));
#12188=CARTESIAN_POINT('Ctrl Pts',(49.1403287769875,10.5381710427577,2.90181519954335));
#12189=CARTESIAN_POINT('Ctrl Pts',(49.12259672862,10.5196372397941,2.92363955400515));
#12190=CARTESIAN_POINT('Ctrl Pts',(49.1059960732651,10.4997217021854,2.94524832138529));
#12191=CARTESIAN_POINT('Ctrl Pts',(49.090663937318,10.4786485987581,2.96644693548253));
#12192=CARTESIAN_POINT('Ctrl Pts',(49.0884574234901,10.4756158775333,2.9694977194893));
#12193=CARTESIAN_POINT('Ctrl Pts',(49.0862772408328,10.4725591253496,2.97254004233701));
#12194=CARTESIAN_POINT('Ctrl Pts',(49.0841238569374,10.4694789537369,2.97557335278404));
#12195=CARTESIAN_POINT('Ctrl Pts',(49.083695781619,10.4688666405089,2.97617635039085));
#12196=CARTESIAN_POINT('Ctrl Pts',(49.0832687102321,10.4682533253048,2.97677906069511));
#12197=CARTESIAN_POINT('Ctrl Pts',(49.0828426468962,10.4676390119166,2.97738147896229));
#12198=CARTESIAN_POINT('',(49.0828426943265,10.4676389273726,-2.97738149942411));
#12199=CARTESIAN_POINT('Origin',(49.0828427124746,0.,-1.66595481168202E-15));
#12200=CARTESIAN_POINT('',(49.3323331704973,10.6616743509686,-2.70149187398906));
#12201=CARTESIAN_POINT('Ctrl Pts',(49.0828426468962,10.4676390119166,-2.97738147896229));
#12202=CARTESIAN_POINT('Ctrl Pts',(49.0832687102357,10.46825332531,-2.97677906068993));
#12203=CARTESIAN_POINT('Ctrl Pts',(49.0836957816155,10.4688666405034,-2.9761763503977));
#12204=CARTESIAN_POINT('Ctrl Pts',(49.0841238569375,10.4694789537365,-2.97557335278547));
#12205=CARTESIAN_POINT('Ctrl Pts',(49.0997803379974,10.4918737755011,-2.95351924171713));
#12206=CARTESIAN_POINT('Ctrl Pts',(49.1168500766551,10.5130338506644,-2.93098701763205));
#12207=CARTESIAN_POINT('Ctrl Pts',(49.1351711977364,10.5327069760909,-2.90819678821397));
#12208=CARTESIAN_POINT('Ctrl Pts',(49.1517839963378,10.5505457136398,-2.88753159585364));
#12209=CARTESIAN_POINT('Ctrl Pts',(49.169426161142,10.5671614160477,-2.86665343070936));
#12210=CARTESIAN_POINT('Ctrl Pts',(49.1880067011391,10.5823374979221,-2.8457516840311));
#12211=CARTESIAN_POINT('Ctrl Pts',(49.1899173698306,10.5838980803649,-2.84360232168846));
#12212=CARTESIAN_POINT('Ctrl Pts',(49.1918379861858,10.5854434157622,-2.84145274014321));
#12213=CARTESIAN_POINT('Ctrl Pts',(49.1937684684827,10.5869732520534,-2.83930316752288));
#12214=CARTESIAN_POINT('Ctrl Pts',(49.209574863942,10.5994992397022,-2.82170290516363));
#12215=CARTESIAN_POINT('Ctrl Pts',(49.2261797406536,10.6111006259049,-2.80395929532978));
#12216=CARTESIAN_POINT('Ctrl Pts',(49.243522871543,10.621520087492,-2.78622125562479));
#12217=CARTESIAN_POINT('Ctrl Pts',(49.2463965558388,10.6232465487248,-2.78328213658884));
#12218=CARTESIAN_POINT('Ctrl Pts',(49.2492905518298,10.6249405188279,-2.78034327008876));
#12219=CARTESIAN_POINT('Ctrl Pts',(49.2522046371122,10.626600777531,-2.77740545786278));
#12220=CARTESIAN_POINT('Ctrl Pts',(49.2692175771233,10.6362936584803,-2.76025399580113));
#12221=CARTESIAN_POINT('Ctrl Pts',(49.2869149560756,10.6448377817445,-2.74313460503217));
#12222=CARTESIAN_POINT('Ctrl Pts',(49.3052032408308,10.6520378277433,-2.7262223666424));
#12223=CARTESIAN_POINT('Ctrl Pts',(49.3141343284223,10.6555539716759,-2.7179632715742));
#12224=CARTESIAN_POINT('Ctrl Pts',(49.3232063992444,10.6587495153119,-2.70975430113892));
#12225=CARTESIAN_POINT('Ctrl Pts',(49.3324087881176,10.6616015016905,-2.70162046046199));
#12226=CARTESIAN_POINT('Ctrl Pts',(49.3323950806311,10.6616812501835,-2.70147713019892));
#12227=CARTESIAN_POINT('Ctrl Pts',(49.317580223994,10.677037679497,-2.63583083212022));
#12228=CARTESIAN_POINT('Ctrl Pts',(49.3037413307877,10.6914388937186,-2.56837430025778));
#12229=CARTESIAN_POINT('Ctrl Pts',(49.2908747206929,10.7048947779706,-2.49999999917371));
#12230=CARTESIAN_POINT('Origin',(48.95,0.,0.));
#12231=CARTESIAN_POINT('',(48.8171572875254,10.1905533656526,2.97937090169063));
#12232=CARTESIAN_POINT('Ctrl Pts',(48.8171572875336,10.1905533656612,2.97937090169057));
#12233=CARTESIAN_POINT('Ctrl Pts',(48.9056698328978,10.2829700356906,2.97869109651476));
#12234=CARTESIAN_POINT('Ctrl Pts',(48.9942328602291,10.3753305077211,2.97802834000757));
#12235=CARTESIAN_POINT('Ctrl Pts',(49.0828426330983,10.4676389975428,2.97738147906302));
#12236=CARTESIAN_POINT('',(48.8171572875336,10.1905533656612,-2.97937090169057));
#12237=CARTESIAN_POINT('Origin',(48.8171572875254,0.,-1.62528346102649E-15));
#12238=CARTESIAN_POINT('Ctrl Pts',(49.0828426330983,10.4676389975428,-2.97738147906302));
#12239=CARTESIAN_POINT('Ctrl Pts',(48.9942328602291,10.3753305077211,-2.97802834000757));
#12240=CARTESIAN_POINT('Ctrl Pts',(48.9056698328978,10.2829700356906,-2.97869109651476));
#12241=CARTESIAN_POINT('Ctrl Pts',(48.8171572875336,10.1905533656612,-2.97937090169057));
#12242=CARTESIAN_POINT('Ctrl Pts',(48.8171572875336,10.1905533656612,2.97937090169057));
#12243=CARTESIAN_POINT('Ctrl Pts',(48.9778062289061,10.3582882347049,2.97813706549952));
#12244=CARTESIAN_POINT('Ctrl Pts',(49.1386214664861,10.5258379779574,2.97695939052998));
#12245=CARTESIAN_POINT('Ctrl Pts',(49.2995806606493,10.6932278010799,2.97583098251121));
#12246=CARTESIAN_POINT('Ctrl Pts',(48.8075014991423,10.1998211785253,2.91326259488353));
#12247=CARTESIAN_POINT('Ctrl Pts',(48.9683243751193,10.3674015107644,2.91210397456444));
#12248=CARTESIAN_POINT('Ctrl Pts',(49.1293028626815,10.5348051777809,2.9109997011877));
#12249=CARTESIAN_POINT('Ctrl Pts',(49.2904188809618,10.7020541703147,2.90994206251764));
#12250=CARTESIAN_POINT('Ctrl Pts',(48.8129307052331,10.1946101212806,2.77448556461726));
#12251=CARTESIAN_POINT('Ctrl Pts',(48.9740100519798,10.3619373600493,2.773609368412));
#12252=CARTESIAN_POINT('Ctrl Pts',(49.1352307428308,10.5291011568935,2.77277138099925));
#12253=CARTESIAN_POINT('Ctrl Pts',(49.2965774530089,10.696121062043,2.77197377859995));
#12254=CARTESIAN_POINT('Ctrl Pts',(48.9060750398012,10.1052083834689,2.5673532928901));
#12255=CARTESIAN_POINT('Ctrl Pts',(49.0671873646562,10.2723851179806,2.56710210511172));
#12256=CARTESIAN_POINT('Ctrl Pts',(49.228440291876,10.4394075522319,2.56686429820521));
#12257=CARTESIAN_POINT('Ctrl Pts',(49.3898161252289,10.6062958341897,2.56663635849247));
#12258=CARTESIAN_POINT('Ctrl Pts',(49.0270075945874,9.98913497324999,2.5));
#12259=CARTESIAN_POINT('Ctrl Pts',(49.1878342329928,10.1564318375549,2.5000050401676));
#12260=CARTESIAN_POINT('Ctrl Pts',(49.3488133909105,10.3235745081665,2.4999954671014));
#12261=CARTESIAN_POINT('Ctrl Pts',(49.509932319593,10.490577063526,2.5));
#12262=CARTESIAN_POINT('Ctrl Pts',(49.1000000000083,9.91907544765526,2.5));
#12263=CARTESIAN_POINT('Ctrl Pts',(49.2606489413807,10.0864495849984,2.5));
#12264=CARTESIAN_POINT('Ctrl Pts',(49.4214641789608,10.2536640921303,2.5));
#12265=CARTESIAN_POINT('Ctrl Pts',(49.582423373124,10.4207398892537,2.5));
#12266=CARTESIAN_POINT('Ctrl Pts',(49.471102006026,10.3051417027149,2.5));
#12267=CARTESIAN_POINT('Ctrl Pts',(49.4519249796202,10.3173672432757,2.49999972617162));
#12268=CARTESIAN_POINT('Ctrl Pts',(49.4342238284002,10.3311503742156,2.50195700947107));
#12269=CARTESIAN_POINT('Ctrl Pts',(49.4181923288807,10.3463856016532,2.50579886168802));
#12270=CARTESIAN_POINT('Ctrl Pts',(49.4094187675144,10.354723387067,2.50790139277969));
#12271=CARTESIAN_POINT('Ctrl Pts',(49.4011454590667,10.363495905895,2.51056922958518));
#12272=CARTESIAN_POINT('Ctrl Pts',(49.3934065141206,10.3726836074799,2.51379620007939));
#12273=CARTESIAN_POINT('Ctrl Pts',(49.3810666011945,10.3873335937945,2.51894167342119));
#12274=CARTESIAN_POINT('Ctrl Pts',(49.3704042965574,10.4026552679914,2.5253725502872));
#12275=CARTESIAN_POINT('Ctrl Pts',(49.3613432382584,10.4184314703273,2.5328774372176));
#12276=CARTESIAN_POINT('Ctrl Pts',(49.3541440763532,10.4309659261399,2.53884019502236));
#12277=CARTESIAN_POINT('Ctrl Pts',(49.3479550864531,10.4437879009631,2.54548197767861));
#12278=CARTESIAN_POINT('Ctrl Pts',(49.342728971544,10.4567969890248,2.55271641212372));
#12279=CARTESIAN_POINT('Ctrl Pts',(49.3360883735995,10.4733270739819,2.56190889475026));
#12280=CARTESIAN_POINT('Ctrl Pts',(49.3310669542557,10.4899794155241,2.57196098389177));
#12281=CARTESIAN_POINT('Ctrl Pts',(49.3275006077779,10.5065537921764,2.58265564561844));
#12282=CARTESIAN_POINT('Ctrl Pts',(49.3247047093136,10.5195475589116,2.5910399090332));
#12283=CARTESIAN_POINT('Ctrl Pts',(49.3228024401235,10.5324940401409,2.59982007462608));
#12284=CARTESIAN_POINT('Ctrl Pts',(49.3217047589493,10.5453062357258,2.60890897643727));
#12285=CARTESIAN_POINT('Ctrl Pts',(49.3210833200784,10.5525597047164,2.61405454785858));
#12286=CARTESIAN_POINT('Ctrl Pts',(49.3207195791288,10.5597703070915,2.61929926750326));
#12287=CARTESIAN_POINT('Ctrl Pts',(49.320593282732,10.5669261888948,2.62462354576028));
#12288=CARTESIAN_POINT('Ctrl Pts',(49.3202452202704,10.5866472094313,2.63929681786496));
#12289=CARTESIAN_POINT('Ctrl Pts',(49.321698592633,10.6065613171611,2.65501534839773));
#12290=CARTESIAN_POINT('Ctrl Pts',(49.3249307613735,10.6265525087281,2.67163246997651));
#12291=CARTESIAN_POINT('Ctrl Pts',(49.3268169984925,10.6382190183124,2.68132993135651));
#12292=CARTESIAN_POINT('Ctrl Pts',(49.3293095351321,10.649911295547,2.69133415471351));
#12293=CARTESIAN_POINT('Ctrl Pts',(49.3324087878956,10.6616015010747,2.70162045999414));
#12294=CARTESIAN_POINT('Origin',(49.1000000000083,9.91907544765526,2.9));
#12295=CARTESIAN_POINT('Ctrl Pts',(49.462305708714,10.3051823273304,2.46082185490775));
#12296=CARTESIAN_POINT('Ctrl Pts',(49.4771037846566,10.3051138491653,2.52723063922477));
#12297=CARTESIAN_POINT('Ctrl Pts',(49.49243661118,10.3050433229319,2.59347917296297));
#12298=CARTESIAN_POINT('Ctrl Pts',(49.5082942562487,10.3049708790319,2.65958704920729));
#12299=CARTESIAN_POINT('Ctrl Pts',(49.4083727211377,10.341288010494,2.47275277189045));
#12300=CARTESIAN_POINT('Ctrl Pts',(49.4232536647421,10.3411829551313,2.53945009831164));
#12301=CARTESIAN_POINT('Ctrl Pts',(49.4386713993083,10.3410740762491,2.60598280249336));
#12302=CARTESIAN_POINT('Ctrl Pts',(49.4546159715293,10.3409629277268,2.67237043888862));
#12303=CARTESIAN_POINT('Ctrl Pts',(49.3031992070178,10.4580767906371,2.49601898654185));
#12304=CARTESIAN_POINT('Ctrl Pts',(49.3182156131681,10.4578563589617,2.56328424053666));
#12305=CARTESIAN_POINT('Ctrl Pts',(49.3337734061097,10.4576291666046,2.63037822823133));
#12306=CARTESIAN_POINT('Ctrl Pts',(49.3498601387948,10.4573959072113,2.69731785735098));
#12307=CARTESIAN_POINT('Ctrl Pts',(49.2766718995763,10.6180800401588,2.50188728935765));
#12308=CARTESIAN_POINT('Ctrl Pts',(49.2916193758389,10.617743529058,2.56932146539533));
#12309=CARTESIAN_POINT('Ctrl Pts',(49.3071014259566,10.6173974045177,2.63657775200008));
#12310=CARTESIAN_POINT('Ctrl Pts',(49.3231160197943,10.6170409930902,2.70368692254473));
#12311=CARTESIAN_POINT('Ctrl Pts',(49.2906111221464,10.7049013470625,2.49880369034412));
#12312=CARTESIAN_POINT('Ctrl Pts',(49.3054535577802,10.7045314987806,2.5661795783969));
#12313=CARTESIAN_POINT('Ctrl Pts',(49.3208320100222,10.7041502377578,2.63338623008397));
#12314=CARTESIAN_POINT('Ctrl Pts',(49.3367364522403,10.7037582059502,2.70044324036495));
#12315=CARTESIAN_POINT('Ctrl Pts',(49.5082942562487,10.3049708790319,-2.65958704920729));
#12316=CARTESIAN_POINT('Ctrl Pts',(49.4924395390992,10.3050433095561,-2.59349137896939));
#12317=CARTESIAN_POINT('Ctrl Pts',(49.4771094475134,10.305113823118,-2.52725510661945));
#12318=CARTESIAN_POINT('Ctrl Pts',(49.4623139056172,10.3051822893992,-2.46085863958849));
#12319=CARTESIAN_POINT('Ctrl Pts',(49.4546159715295,10.3409629277267,-2.67237043888858));
#12320=CARTESIAN_POINT('Ctrl Pts',(49.4386743432776,10.3410740557268,-2.60599506015401));
#12321=CARTESIAN_POINT('Ctrl Pts',(49.4232593589763,10.3411829150475,-2.53947467065603));
#12322=CARTESIAN_POINT('Ctrl Pts',(49.4083809639253,10.3412879521802,-2.47278971640008));
#12323=CARTESIAN_POINT('Ctrl Pts',(49.3498601387952,10.4573959072108,-2.69731785735089));
#12324=CARTESIAN_POINT('Ctrl Pts',(49.3337763763275,10.4576291235356,-2.6303905878106));
#12325=CARTESIAN_POINT('Ctrl Pts',(49.3182213589273,10.4578562750788,-2.56330901994368));
#12326=CARTESIAN_POINT('Ctrl Pts',(49.3032075250344,10.4580766685106,-2.49605624588246));
#12327=CARTESIAN_POINT('Ctrl Pts',(49.3231160197944,10.6170409930891,-2.7036869225447));
#12328=CARTESIAN_POINT('Ctrl Pts',(49.3071043828546,10.6173973387096,-2.63659014288315));
#12329=CARTESIAN_POINT('Ctrl Pts',(49.2916250945902,10.6177434011025,-2.56934630598959));
#12330=CARTESIAN_POINT('Ctrl Pts',(49.2766801784892,10.6180798538746,-2.50192464095437));
#12331=CARTESIAN_POINT('Ctrl Pts',(49.3367364522401,10.7037582059489,-2.700443240365));
#12332=CARTESIAN_POINT('Ctrl Pts',(49.3208349465817,10.7041501653727,-2.63339861133636));
#12333=CARTESIAN_POINT('Ctrl Pts',(49.3054592374878,10.7045313579687,-2.56620439965167));
#12334=CARTESIAN_POINT('Ctrl Pts',(49.2906193436209,10.7049011421962,-2.49884101071544));
#12335=CARTESIAN_POINT('',(49.4711020394073,10.3051416724427,-2.5));
#12336=CARTESIAN_POINT('Ctrl Pts',(49.3323950805385,10.6616812492885,-2.70147713001029));
#12337=CARTESIAN_POINT('Ctrl Pts',(49.3271569720922,10.6417619720421,-2.68393641922588));
#12338=CARTESIAN_POINT('Ctrl Pts',(49.3237005583529,10.6218293402928,-2.66722269704707));
#12339=CARTESIAN_POINT('Ctrl Pts',(49.3219885926706,10.6020145351385,-2.65145685176126));
#12340=CARTESIAN_POINT('Ctrl Pts',(49.3209757435438,10.5902915150407,-2.64212931511863));
#12341=CARTESIAN_POINT('Ctrl Pts',(49.3205744428189,10.5786096190675,-2.63313320519147));
#12342=CARTESIAN_POINT('Ctrl Pts',(49.3207850049258,10.5669968946579,-2.62449066979262));
#12343=CARTESIAN_POINT('Ctrl Pts',(49.3210756127816,10.550969561956,-2.6125626514104));
#12344=CARTESIAN_POINT('Ctrl Pts',(49.3225361848226,10.5346775925373,-2.60100536084123));
#12345=CARTESIAN_POINT('Ctrl Pts',(49.3253648341183,10.5182626775943,-2.59003870410598));
#12346=CARTESIAN_POINT('Ctrl Pts',(49.3280417284346,10.5027284109103,-2.57966040053581));
#12347=CARTESIAN_POINT('Ctrl Pts',(49.331943942577,10.4870838027976,-2.56981112723947));
#12348=CARTESIAN_POINT('Ctrl Pts',(49.3372505335242,10.4714944194039,-2.5606726536798));
#12349=CARTESIAN_POINT('Ctrl Pts',(49.338907744272,10.466625965444,-2.55781877314679));
#12350=CARTESIAN_POINT('Ctrl Pts',(49.3407019993306,10.4617632603077,-2.55503417504958));
#12351=CARTESIAN_POINT('Ctrl Pts',(49.3426389695942,10.4569123869465,-2.55232427803795));
#12352=CARTESIAN_POINT('Ctrl Pts',(49.3436752717814,10.4543171118569,-2.55087445082417));
#12353=CARTESIAN_POINT('Ctrl Pts',(49.3447507774767,10.451729479217,-2.54944858395426));
#12354=CARTESIAN_POINT('Ctrl Pts',(49.3458660878379,10.4491502726166,-2.54804741897205));
#12355=CARTESIAN_POINT('Ctrl Pts',(49.3528539912289,10.4329904240435,-2.53926851233641));
#12356=CARTESIAN_POINT('Ctrl Pts',(49.3614046849159,10.4171575527942,-2.5314598314099));
#12357=CARTESIAN_POINT('Ctrl Pts',(49.3715767266835,10.4018302197805,-2.52481994804416));
#12358=CARTESIAN_POINT('Ctrl Pts',(49.3781479620868,10.3919286173649,-2.52053052045005));
#12359=CARTESIAN_POINT('Ctrl Pts',(49.385395823602,10.3822388736403,-2.51672872957607));
#12360=CARTESIAN_POINT('Ctrl Pts',(49.3933348932719,10.3728207109584,-2.51346660440115));
#12361=CARTESIAN_POINT('Ctrl Pts',(49.4070771902143,10.3565181473573,-2.50781996132063));
#12362=CARTESIAN_POINT('Ctrl Pts',(49.4224925047283,10.3414985031374,-2.50395905075391));
#12363=CARTESIAN_POINT('Ctrl Pts',(49.4393853211129,10.327896747852,-2.50186576538707));
#12364=CARTESIAN_POINT('Ctrl Pts',(49.4494441471084,10.3197975838917,-2.50061931880381));
#12365=CARTESIAN_POINT('Ctrl Pts',(49.4600277835471,10.3122015103339,-2.49999924910275));
#12366=CARTESIAN_POINT('Ctrl Pts',(49.4711018430278,10.3051416733453,-2.49999916367266));
#12367=CARTESIAN_POINT('Ctrl Pts',(49.2908747205623,10.7048947773287,-2.499999999072));
#12368=CARTESIAN_POINT('Ctrl Pts',(49.2872058781153,10.6831077488647,-2.49999977996358));
#12369=CARTESIAN_POINT('Ctrl Pts',(49.2854473079225,10.6610039750184,-2.49998517158562));
#12370=CARTESIAN_POINT('Ctrl Pts',(49.2855726481819,10.6388034196963,-2.49997268059858));
#12371=CARTESIAN_POINT('Ctrl Pts',(49.2856981913103,10.6165669317439,-2.49996016939429));
#12372=CARTESIAN_POINT('Ctrl Pts',(49.2877121963881,10.5944414635718,-2.49994942515778));
#12373=CARTESIAN_POINT('Ctrl Pts',(49.2915330177167,10.5726477963842,-2.49994809325073));
#12374=CARTESIAN_POINT('Ctrl Pts',(49.2953838688655,10.5506828414414,-2.49994675087554));
#12375=CARTESIAN_POINT('Ctrl Pts',(49.3010702648263,10.5290535111454,-2.49995491240654));
#12376=CARTESIAN_POINT('Ctrl Pts',(49.3085583741435,10.5079899006643,-2.49996733309932));
#12377=CARTESIAN_POINT('Ctrl Pts',(49.3107658785906,10.5017803206703,-2.49997099473584));
#12378=CARTESIAN_POINT('Ctrl Pts',(49.3131302814176,10.4956200105166,-2.49997494360772));
#12379=CARTESIAN_POINT('Ctrl Pts',(49.3156514926051,10.4895152119484,-2.49997884080595));
#12380=CARTESIAN_POINT('Ctrl Pts',(49.3213480167851,10.4757217888387,-2.49998764628964));
#12381=CARTESIAN_POINT('Ctrl Pts',(49.3278098816835,10.4622952988396,-2.49999625392971));
#12382=CARTESIAN_POINT('Ctrl Pts',(49.3350146013469,10.4492980432451,-2.50000038352441));
#12383=CARTESIAN_POINT('Ctrl Pts',(49.3458363826384,10.4297756379321,-2.50000658634322));
#12384=CARTESIAN_POINT('Ctrl Pts',(49.3583318951607,10.4112200704296,-2.50000320120766));
#12385=CARTESIAN_POINT('Ctrl Pts',(49.3723085264239,10.393783414394,-2.50000070356517));
#12386=CARTESIAN_POINT('Ctrl Pts',(49.3817076056388,10.3820575193457,-2.49999902393729));
#12387=CARTESIAN_POINT('Ctrl Pts',(49.3917776159901,10.3708379724724,-2.49999747922745));
#12388=CARTESIAN_POINT('Ctrl Pts',(49.4024704737568,10.3601786152418,-2.49999676540344));
#12389=CARTESIAN_POINT('Ctrl Pts',(49.4184910300295,10.3442082510913,-2.49999569591783));
#12390=CARTESIAN_POINT('Ctrl Pts',(49.4357738390234,10.3296276305099,-2.49999714156594));
#12391=CARTESIAN_POINT('Ctrl Pts',(49.4541233624076,10.3165800826316,-2.499998440249));
#12392=CARTESIAN_POINT('Ctrl Pts',(49.4596860976899,10.3126246635502,-2.49999883395024));
#12393=CARTESIAN_POINT('Ctrl Pts',(49.4653471679471,10.308810334878,-2.49999915006047));
#12394=CARTESIAN_POINT('Ctrl Pts',(49.4711018430278,10.3051416733453,-2.49999916367266));
#12395=CARTESIAN_POINT('Ctrl Pts',(49.2995806606493,10.6932278010799,-2.97583098251121));
#12396=CARTESIAN_POINT('Ctrl Pts',(49.1386214664862,10.5258379779574,-2.97695939052998));
#12397=CARTESIAN_POINT('Ctrl Pts',(48.9778062289061,10.3582882347048,-2.97813706549952));
#12398=CARTESIAN_POINT('Ctrl Pts',(48.8171572875336,10.1905533656612,-2.97937090169057));
#12399=CARTESIAN_POINT('Ctrl Pts',(49.2904188809618,10.7020541703147,-2.90994206251764));
#12400=CARTESIAN_POINT('Ctrl Pts',(49.1293028626815,10.534805177781,-2.9109997011877));
#12401=CARTESIAN_POINT('Ctrl Pts',(48.9683243751193,10.3674015107643,-2.91210397456444));
#12402=CARTESIAN_POINT('Ctrl Pts',(48.8075014991423,10.1998211785253,-2.91326259488353));
#12403=CARTESIAN_POINT('Ctrl Pts',(49.2965774530089,10.696121062043,-2.77197377859995));
#12404=CARTESIAN_POINT('Ctrl Pts',(49.1352307428308,10.5291011568935,-2.77277138099925));
#12405=CARTESIAN_POINT('Ctrl Pts',(48.9740100519798,10.3619373600493,-2.773609368412));
#12406=CARTESIAN_POINT('Ctrl Pts',(48.8129307052331,10.1946101212806,-2.77448556461726));
#12407=CARTESIAN_POINT('Ctrl Pts',(49.3898161252289,10.6062958341897,-2.56663635849247));
#12408=CARTESIAN_POINT('Ctrl Pts',(49.228440291876,10.439407552232,-2.5668642982052));
#12409=CARTESIAN_POINT('Ctrl Pts',(49.0671873646562,10.2723851179806,-2.56710210511172));
#12410=CARTESIAN_POINT('Ctrl Pts',(48.9060750398012,10.1052083834689,-2.5673532928901));
#12411=CARTESIAN_POINT('Ctrl Pts',(49.509932319593,10.490577063526,-2.5));
#12412=CARTESIAN_POINT('Ctrl Pts',(49.3488133909105,10.3235745081665,-2.4999954671014));
#12413=CARTESIAN_POINT('Ctrl Pts',(49.1878342329928,10.1564318375549,-2.50000504016761));
#12414=CARTESIAN_POINT('Ctrl Pts',(49.0270075945874,9.98913497324999,-2.5));
#12415=CARTESIAN_POINT('Ctrl Pts',(49.582423373124,10.4207398892537,-2.5));
#12416=CARTESIAN_POINT('Ctrl Pts',(49.4214641789608,10.2536640921303,-2.5));
#12417=CARTESIAN_POINT('Ctrl Pts',(49.2606489413807,10.0864495849984,-2.5));
#12418=CARTESIAN_POINT('Ctrl Pts',(49.1000000000083,9.91907544765526,-2.5));
#12419=CARTESIAN_POINT('',(49.1000000000041,9.91907544765526,-2.5));
#12420=CARTESIAN_POINT('Origin',(49.1000000000083,9.91907544765526,-2.9));
#12421=CARTESIAN_POINT('Ctrl Pts',(49.1000000000083,9.91907544765526,-2.5));
#12422=CARTESIAN_POINT('Ctrl Pts',(49.2236056134068,10.0478555238674,-2.5));
#12423=CARTESIAN_POINT('Ctrl Pts',(49.3473096739212,10.176541099224,-2.5));
#12424=CARTESIAN_POINT('Ctrl Pts',(49.471102006026,10.3051417027149,-2.5));
#12425=CARTESIAN_POINT('Origin',(49.1,0.,0.));
#12426=CARTESIAN_POINT('',(48.7,9.91907544764665,2.9));
#12427=CARTESIAN_POINT('Origin',(49.1,9.91907544764666,2.9));
#12428=CARTESIAN_POINT('',(48.7,9.91907544764665,-2.9));
#12429=CARTESIAN_POINT('Origin',(48.7,0.,0.));
#12430=CARTESIAN_POINT('Origin',(49.1,9.91907544764666,-2.9));
#12431=CARTESIAN_POINT('Origin',(49.1,9.91907544764666,-2.9));
#12432=CARTESIAN_POINT('Origin',(49.1,9.91907544764666,-2.9));
#12433=CARTESIAN_POINT('Origin',(49.1,9.91907544764666,2.9));
#12434=CARTESIAN_POINT('Origin',(49.1,9.91907544764666,2.9));
#12435=CARTESIAN_POINT('Origin',(58.5,8.62,-2.5));
#12436=CARTESIAN_POINT('',(69.,10.24,-2.5));
#12437=CARTESIAN_POINT('',(49.1,7.83022988168291,-2.5));
#12438=CARTESIAN_POINT('',(49.1,9.56,-2.5));
#12439=CARTESIAN_POINT('',(69.0218379181362,7.83022988168291,-2.5));
#12440=CARTESIAN_POINT('',(59.6,7.83022988168291,-2.5));
#12441=CARTESIAN_POINT('',(69.,7.9669630349337,-2.5));
#12442=CARTESIAN_POINT('Ctrl Pts',(69.,7.96696303493369,-2.5));
#12443=CARTESIAN_POINT('Ctrl Pts',(69.,7.92356314245502,-2.5));
#12444=CARTESIAN_POINT('Ctrl Pts',(69.0075947074924,7.87360329207051,-2.5));
#12445=CARTESIAN_POINT('Ctrl Pts',(69.0218379181362,7.83022988168291,-2.5));
#12446=CARTESIAN_POINT('',(69.,10.24,-2.5));
#12447=CARTESIAN_POINT('',(69.,7.,-2.5));
#12448=CARTESIAN_POINT('',(69.,10.24,-2.5));
#12449=CARTESIAN_POINT('Origin',(49.1,9.56,-2.9));
#12450=CARTESIAN_POINT('',(48.7,7.83022988168291,-2.9));
#12451=CARTESIAN_POINT('',(48.7,9.56,-2.9));
#12452=CARTESIAN_POINT('Origin',(49.1,7.83022988168291,-2.9));
#12453=CARTESIAN_POINT('Origin',(48.7,10.5,0.));
#12454=CARTESIAN_POINT('',(48.7,7.83022988168291,2.9));
#12455=CARTESIAN_POINT('',(48.7,9.56,2.9));
#12456=CARTESIAN_POINT('Origin',(48.7,0.,0.));
#12457=CARTESIAN_POINT('Origin',(49.1,9.56,2.9));
#12458=CARTESIAN_POINT('Origin',(49.1,7.83022988168291,2.9));
#12459=CARTESIAN_POINT('Origin',(70.1,0.,0.));
#12460=CARTESIAN_POINT('',(70.5,-1.26558852657178E-15,10.3343145750508));
#12461=CARTESIAN_POINT('Origin',(70.5,0.,0.));
#12462=CARTESIAN_POINT('Origin',(70.1,-1.26558852657178E-15,10.3343145750508));
#12463=CARTESIAN_POINT('Origin',(70.5,7.95,0.));
#12464=CARTESIAN_POINT('',(70.5,-1.02258007728804E-15,8.35));
#12465=CARTESIAN_POINT('Origin',(70.5,0.,0.));
#12466=CARTESIAN_POINT('Origin',(70.1,0.,0.));
#12467=CARTESIAN_POINT('',(70.1,-9.73594205322146E-16,7.95));
#12468=CARTESIAN_POINT('',(70.1,-7.95,-9.73594205322146E-16));
#12469=CARTESIAN_POINT('Origin',(70.1,0.,0.));
#12470=CARTESIAN_POINT('Origin',(70.1,0.,0.));
#12471=CARTESIAN_POINT('Origin',(70.1,-1.02258007728804E-15,8.35));
#12472=CARTESIAN_POINT('Origin',(59.6,0.,0.));
#12473=CARTESIAN_POINT('',(49.1,-7.95,-9.73594205322146E-16));
#12474=CARTESIAN_POINT('',(59.6,-7.95,-9.73594205322146E-16));
#12475=CARTESIAN_POINT('',(49.1,7.45512904902744,2.76107784431138));
#12476=CARTESIAN_POINT('Origin',(49.1,0.,0.));
#12477=CARTESIAN_POINT('',(69.4,7.45512904902744,2.76107784431138));
#12478=CARTESIAN_POINT('',(59.6,7.45512904902744,2.76107784431138));
#12479=CARTESIAN_POINT('',(69.4,7.45512904902744,-2.76107784431138));
#12480=CARTESIAN_POINT('Origin',(69.4,0.,0.));
#12481=CARTESIAN_POINT('',(49.1,7.45512904902744,-2.76107784431138));
#12482=CARTESIAN_POINT('',(59.6,7.45512904902744,-2.76107784431138));
#12483=CARTESIAN_POINT('Origin',(49.1,0.,0.));
#12484=CARTESIAN_POINT('Origin',(69.,10.24,0.));
#12485=CARTESIAN_POINT('',(69.,10.24,0.));
#12486=CARTESIAN_POINT('Origin',(49.1,7.83022988168291,-2.9));
#12487=CARTESIAN_POINT('Origin',(49.1,7.83022988168291,-2.9));
#12488=CARTESIAN_POINT('Origin',(49.1,7.83022988168291,-2.9));
#12489=CARTESIAN_POINT('Origin',(49.1,7.83022988168291,2.9));
#12490=CARTESIAN_POINT('Origin',(49.1,7.83022988168291,2.9));
#12491=CARTESIAN_POINT('Origin',(49.1,7.83022988168291,2.9));
#12492=CARTESIAN_POINT('Origin',(49.1,0.,0.));
#12493=CARTESIAN_POINT('Origin',(59.6,7.83022988168291,-2.9));
#12494=CARTESIAN_POINT('Ctrl Pts',(69.4,7.45512904902744,-2.76107784431138));
#12495=CARTESIAN_POINT('Ctrl Pts',(69.3990583301394,7.45544816645284,-2.76021620196651));
#12496=CARTESIAN_POINT('Ctrl Pts',(69.3981166569032,7.45577025393396,-2.75935565609771));
#12497=CARTESIAN_POINT('Ctrl Pts',(69.3240866264373,7.48132475515606,-2.69178981004436));
#12498=CARTESIAN_POINT('Ctrl Pts',(69.2523194411631,7.52398051258273,-2.6328664623909));
#12499=CARTESIAN_POINT('Ctrl Pts',(69.142314610906,7.62274186069682,-2.55365184512958));
#12500=CARTESIAN_POINT('Ctrl Pts',(69.1013968001416,7.67221396448289,-2.52842397830978));
#12501=CARTESIAN_POINT('Ctrl Pts',(69.0504474618219,7.75813083757979,-2.50509269239044));
#12502=CARTESIAN_POINT('Ctrl Pts',(69.0339490479658,7.79334908159564,-2.5));
#12503=CARTESIAN_POINT('Ctrl Pts',(69.0218379181362,7.83022988168291,-2.5));
#12504=CARTESIAN_POINT('Origin',(69.4,0.,0.));
#12505=CARTESIAN_POINT('Ctrl Pts',(69.4,7.45512904902744,2.76107784431138));
#12506=CARTESIAN_POINT('Ctrl Pts',(69.3990583301394,7.45544816645284,2.76021620196653));
#12507=CARTESIAN_POINT('Ctrl Pts',(69.3981166569034,7.45577025393397,2.75935565609769));
#12508=CARTESIAN_POINT('Ctrl Pts',(69.3240866264303,7.481324755157,2.69178981004185));
#12509=CARTESIAN_POINT('Ctrl Pts',(69.2523194411595,7.52398051258612,2.6328664623884));
#12510=CARTESIAN_POINT('Ctrl Pts',(69.1423146109063,7.62274186069636,2.55365184512979));
#12511=CARTESIAN_POINT('Ctrl Pts',(69.1013968001419,7.67221396448251,2.52842397830999));
#12512=CARTESIAN_POINT('Ctrl Pts',(69.0504474618222,7.75813083757931,2.50509269239052));
#12513=CARTESIAN_POINT('Ctrl Pts',(69.0339490479659,7.79334908159538,2.5));
#12514=CARTESIAN_POINT('Ctrl Pts',(69.0218379181362,7.83022988168291,2.5));
#12515=CARTESIAN_POINT('Origin',(69.,0.,0.));
#12516=CARTESIAN_POINT('Origin',(59.6,7.83022988168291,2.9));
#12517=CARTESIAN_POINT('Origin',(69.,7.,0.));
#12795=UNCERTAINTY_MEASURE_WITH_UNIT(LENGTH_MEASURE(0.01),#12814,
'DISTANCE_ACCURACY_VALUE',
'Maximum model space distance between geometric entities at asserted c
onnectivities');
#12801=UNCERTAINTY_MEASURE_WITH_UNIT(LENGTH_MEASURE(0.01),#12814,
'DISTANCE_ACCURACY_VALUE',
'Maximum model space distance between geometric entities at asserted c
onnectivities');
#12807=(
GEOMETRIC_REPRESENTATION_CONTEXT(3)
GLOBAL_UNCERTAINTY_ASSIGNED_CONTEXT((#12795))
GLOBAL_UNIT_ASSIGNED_CONTEXT((#12814,#12816,#12817))
REPRESENTATION_CONTEXT('','3D')
);
#12813=(
GEOMETRIC_REPRESENTATION_CONTEXT(3)
GLOBAL_UNCERTAINTY_ASSIGNED_CONTEXT((#12801))
GLOBAL_UNIT_ASSIGNED_CONTEXT((#12814,#12816,#12817))
REPRESENTATION_CONTEXT('','3D')
);
#12814=(
LENGTH_UNIT()
NAMED_UNIT(*)
SI_UNIT(.MILLI.,.METRE.)
);
#12816=(
NAMED_UNIT(*)
PLANE_ANGLE_UNIT()
SI_UNIT($,.RADIAN.)
);
#12817=(
NAMED_UNIT(*)
SI_UNIT($,.STERADIAN.)
SOLID_ANGLE_UNIT()
);
#12823=SHAPE_DEFINITION_REPRESENTATION(#12834,#12858);
#12834=PRODUCT_DEFINITION_SHAPE('',$,#12870);
#12858=SHAPE_REPRESENTATION('',(#4796),#12807);
#12864=PRODUCT_DEFINITION_CONTEXT('part definition',#12899,'design');
#12870=PRODUCT_DEFINITION('2026-10-11-12-17-35-869',
'05_Upper_Sheave_Hub',#12881,#12864);
#12881=PRODUCT_DEFINITION_FORMATION('',$,#12906);
#12899=APPLICATION_CONTEXT(
'Core Data for Automotive Mechanical Design Process');
#12900=PRODUCT_CONTEXT('part definition',#12899,'mechanical');
#12906=PRODUCT('2026-10-11-12-17-35-869','05_Upper_Sheave_Hub',$,(#12900));
#12954=COLOUR_RGB('Light Blue',0.38,0.62,0.78);
#12955=FILL_AREA_STYLE_COLOUR('',#12954);
#12956=FILL_AREA_STYLE('',(#12955));
#12957=SURFACE_STYLE_FILL_AREA(#12956);
#12958=SURFACE_SIDE_STYLE('',(#12957));
#12959=SURFACE_STYLE_USAGE(.BOTH.,#12958);
#12960=PRESENTATION_STYLE_ASSIGNMENT((#12959));
ENDSEC;
END-ISO-10303-21;
